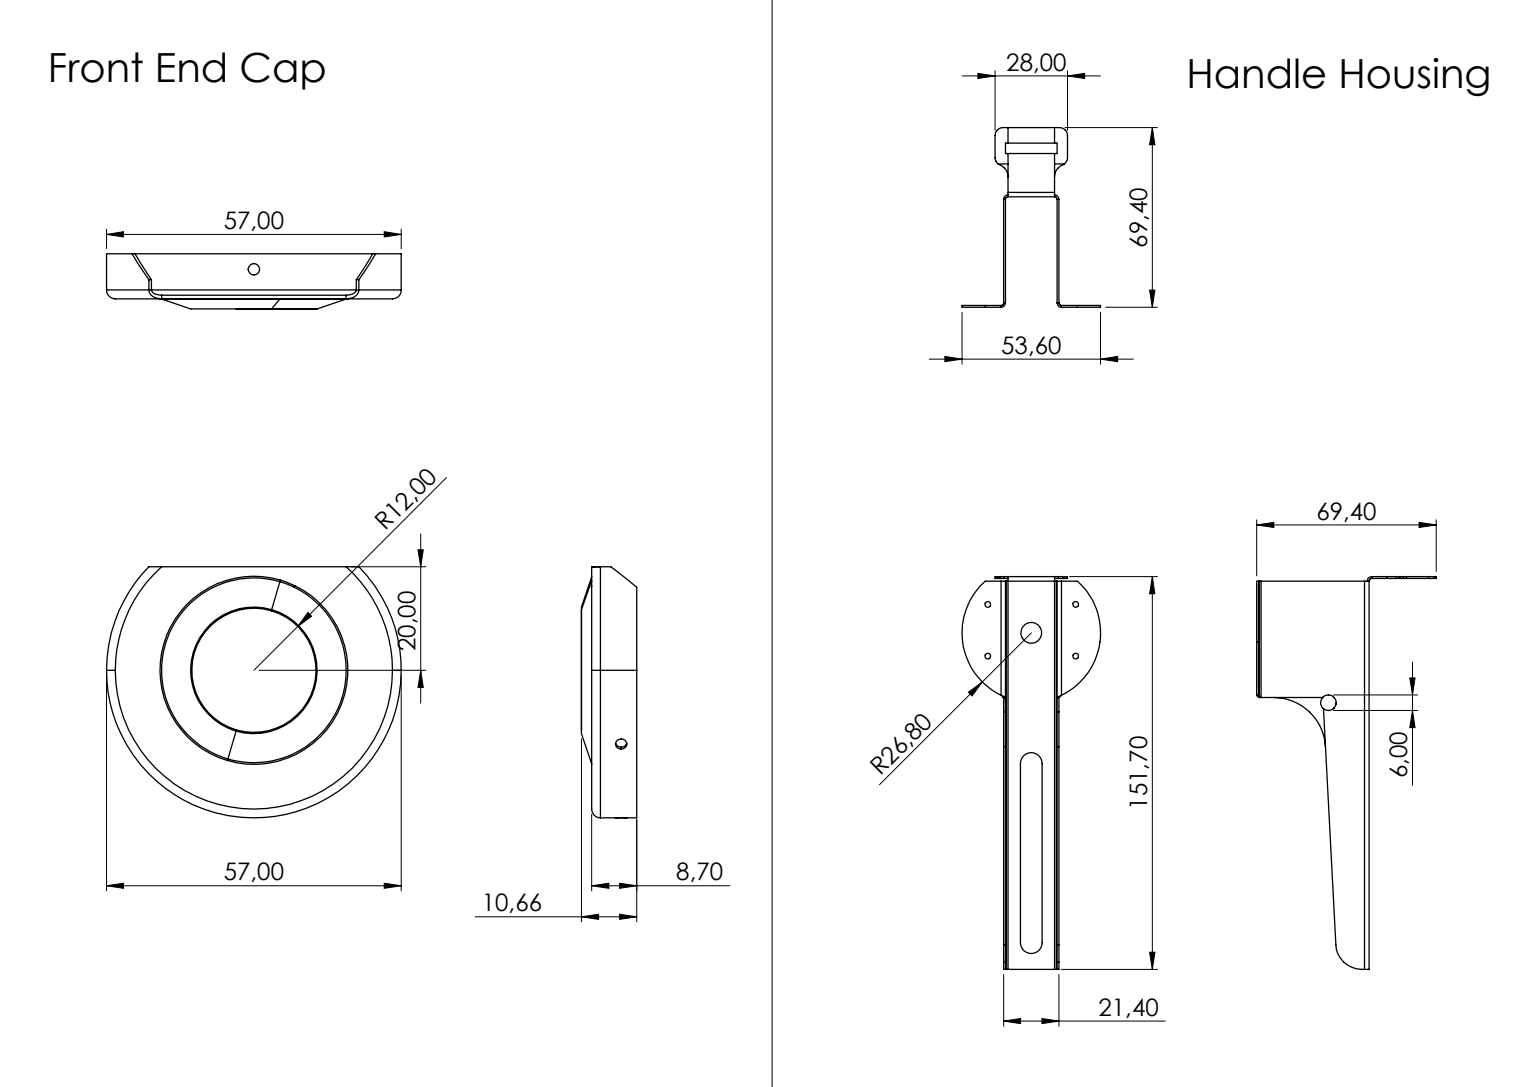
ISO-10303-21;
HEADER;
FILE_DESCRIPTION (('STEP AP214'),
    '1' );
FILE_NAME ('Front End Cap.step',
    '2026-10-06T09:00:30',
    ( '' ),
    ( '' ),
    'SwSTEP 2.0',
    'SolidWorks 2020',
    '' );
FILE_SCHEMA (( 'AUTOMOTIVE_DESIGN' ));
ENDSEC;

DATA;
#20=CARTESIAN_POINT ( 'NONE',  ( -0.8259893079150000261, -28.48844349870000059, 224.2403608809999866 ) ) ;
#22=CARTESIAN_POINT ( 'NONE',  ( 24.25874038310000103, -14.95904359230000047, 225.7601370010000039 ) ) ;
#50=EDGE_CURVE ( 'NONE', #6418, #21281, #18108, .T. ) ;
#55=VERTEX_POINT ( 'NONE', #6316 ) ;
#63=CARTESIAN_POINT ( 'NONE',  ( 24.57933163011563238, -12.98840299560160538, 225.3593307347778136 ) ) ;
#67=CARTESIAN_POINT ( 'NONE',  ( 1.127732790480000080, -28.47784299079999926, 225.0000014190000002 ) ) ;
#70=EDGE_CURVE ( 'NONE', #662, #13739, #1640, .T. ) ;
#83=CARTESIAN_POINT ( 'NONE',  ( 27.71720220739999974, -1.975806291350000238E-11, 229.4485730569999760 ) ) ;
#84=CARTESIAN_POINT ( 'NONE',  ( -11.57541201399999942, -14.20905793120000027, 230.6999999999999886 ) ) ;
#86=CARTESIAN_POINT ( 'NONE',  ( 25.26810488179999936, 12.77004255139999955, 229.0000000000000000 ) ) ;
#91=CARTESIAN_POINT ( 'NONE',  ( 20.67177784749999958, 17.22892977999999786, 230.6999999999999886 ) ) ;
#104=CARTESIAN_POINT ( 'NONE',  ( 24.55806919409999978, -14.46257963250000067, 223.9201486480000085 ) ) ;
#111=CARTESIAN_POINT ( 'NONE',  ( 24.34123158960000310, -14.82477075290000101, 225.9012998019999827 ) ) ;
#112=CARTESIAN_POINT ( 'NONE',  ( -12.01652311039999965, 1.520041121179999788, 231.9999989789999972 ) ) ;
#117=CARTESIAN_POINT ( 'NONE',  ( 24.40260331739102639, -13.31784478726558163, 224.1134674150510477 ) ) ;
#138=CARTESIAN_POINT ( 'NONE',  ( 28.49999999979999998, 4.443028818220000176, 229.0000000000000000 ) ) ;
#140=CARTESIAN_POINT ( 'NONE',  ( 5.010073463369999480, 11.17224087250000153, 232.6627648150000027 ) ) ;
#199=ORIENTED_EDGE ( 'NONE', *, *, #6289, .F. ) ;
#200=CARTESIAN_POINT ( 'NONE',  ( 25.11738521000000190, -13.46751580659999981, 225.6806823370000075 ) ) ;
#209=CARTESIAN_POINT ( 'NONE',  ( -5.361385120510000490, 31.61859227569999931, 222.0000000000000000 ) ) ;
#217=CARTESIAN_POINT ( 'NONE',  ( 24.50095082274352265, -13.13603084652294051, 225.6822660555842219 ) ) ;
#235=CARTESIAN_POINT ( 'NONE',  ( 21.99374050320000151, 17.63454380109999775, 229.1414208810000162 ) ) ;
#239=CARTESIAN_POINT ( 'NONE',  ( 22.83443070970000122, 16.43389729289999934, 229.0000000010000178 ) ) ;
#270=CARTESIAN_POINT ( 'NONE',  ( -26.95773186790000153, 8.656139628340000058, 223.3999999999999773 ) ) ;
#280=CARTESIAN_POINT ( 'NONE',  ( 23.65332633301680687, -14.60697862033088512, 225.7326966119605061 ) ) ;
#285=ORIENTED_EDGE ( 'NONE', *, *, #4802, .T. ) ;
#289=CARTESIAN_POINT ( 'NONE',  ( -24.87138426050000106, -13.91768300640000078, 223.9574921340000060 ) ) ;
#292=CARTESIAN_POINT ( 'NONE',  ( 24.30716200859999887, -13.49132717699999873, 226.0027513979999867 ) ) ;
#302=CARTESIAN_POINT ( 'NONE',  ( 8.575788938069999645, 8.809323376420000073, 232.6627648150000027 ) ) ;
#306=CARTESIAN_POINT ( 'NONE',  ( 28.49999999970000175, -7.466149220240000162, 229.2404163060000144 ) ) ;
#319=CARTESIAN_POINT ( 'NONE',  ( -24.34385441500000269, 13.50419739129999996, 229.9172023120000006 ) ) ;
#333=CARTESIAN_POINT ( 'NONE',  ( -0.07056952541350000607, -28.50017087330000010, 223.9013489249999793 ) ) ;
#354=B_SPLINE_SURFACE_WITH_KNOTS ( 'NONE', 5, 1, ( 
 ( #10886, #5534 ),
 ( #25047, #15138 ),
 ( #29454, #22387 ),
 ( #22540, #832 ),
 ( #10575, #22684 ),
 ( #7887, #24739 ) ),
 .UNSPECIFIED., .F., .F., .F.,
 ( 6, 6 ),
 ( 2, 2 ),
 ( 0.000000000000000000, 2.000000000000000000 ),
 ( 4.440892098500000003E-16, 0.7000000000030000002 ),
 .UNSPECIFIED. ) ;
#379=ORIENTED_EDGE ( 'NONE', *, *, #13979, .T. ) ;
#392=CARTESIAN_POINT ( 'NONE',  ( 25.84472112319999937, 9.051226241580000220, 230.0000000000000000 ) ) ;
#406=ORIENTED_EDGE ( 'NONE', *, *, #23149, .F. ) ;
#426=CARTESIAN_POINT ( 'NONE',  ( -7.523368333400000552, -9.723541495030000092, 232.6627643349999914 ) ) ;
#429=CARTESIAN_POINT ( 'NONE',  ( -6.304462755850305911, -10.33059293845434645, 232.0000000000046043 ) ) ;
#433=B_SPLINE_CURVE_WITH_KNOTS ( 'NONE', 5,
 ( #4051, #25135, #25459, #5930, #17879, #25619 ),
 .UNSPECIFIED., .F., .F.,
 ( 6, 6 ),
 ( -7.000000000120000010, -4.999999893120000038 ),
 .UNSPECIFIED. ) ;
#444=CARTESIAN_POINT ( 'NONE',  ( -24.26052213770000066, -13.57583965319999919, 223.9574921340000060 ) ) ;
#453=VERTEX_POINT ( 'NONE', #9877 ) ;
#456=CARTESIAN_POINT ( 'NONE',  ( -24.82465127917437542, -14.00098045660550916, 223.9261769685532784 ) ) ;
#457=CARTESIAN_POINT ( 'NONE',  ( 10.59650700230000098, -5.774382186429999564, 231.9999991140000191 ) ) ;
#466=ADVANCED_FACE ( 'NONE', ( #21379 ), #11165, .F. ) ;
#477=CARTESIAN_POINT ( 'NONE',  ( -26.13021838950000131, 9.136631768579999147, 229.9751247030000059 ) ) ;
#484=ORIENTED_EDGE ( 'NONE', *, *, #3647, .F. ) ;
#488=CARTESIAN_POINT ( 'NONE',  ( 18.64708650441101767, 19.99999271436163539, 230.6104614892431073 ) ) ;
#495=CARTESIAN_POINT ( 'NONE',  ( -20.30396347049999761, 20.00000000670000233, 227.0000000000000000 ) ) ;
#508=CARTESIAN_POINT ( 'NONE',  ( 1.015231355570000105, -28.48218680760000154, 225.5064715119999903 ) ) ;
#529=FACE_OUTER_BOUND ( 'NONE', #18862, .T. ) ;
#532=EDGE_CURVE ( 'NONE', #10448, #2003, #10192, .T. ) ;
#543=CARTESIAN_POINT ( 'NONE',  ( -0.9721910944845530977, -28.48371442619422567, 224.4394323450521540 ) ) ;
#551=CARTESIAN_POINT ( 'NONE',  ( 26.78508784419999955, 9.380747199480000020, 229.2930777859999978 ) ) ;
#552=CARTESIAN_POINT ( 'NONE',  ( -10.87631678760000042, 14.78838196149999895, 230.6999999999999886 ) ) ;
#560=ADVANCED_FACE ( 'NONE', ( #602, #27628 ), #17709, .F. ) ;
#595=CARTESIAN_POINT ( 'NONE',  ( 24.19477113890000197, -13.69187437440000110, 226.0798554400000171 ) ) ;
#602=FACE_BOUND ( 'NONE', #30223, .T. ) ;
#606=CARTESIAN_POINT ( 'NONE',  ( 11.05434102880000147, 5.380509146490000560, 232.6627648150000027 ) ) ;
#627=CARTESIAN_POINT ( 'NONE',  ( -18.03440174900000059, 20.21871556809999859, 229.9751246760000072 ) ) ;
#630=B_SPLINE_CURVE_WITH_KNOTS ( 'NONE', 1,
 ( #19801, #8283 ),
 .UNSPECIFIED., .F., .F.,
 ( 2, 2 ),
 ( -2.557291473029999731E-06, 0.7000000000009999335 ),
 .UNSPECIFIED. ) ;
#631=B_SPLINE_CURVE_WITH_KNOTS ( 'NONE', 5,
 ( #31112, #6871, #7037, #18836, #26396, #16473, #11758, #23732, #2168 ),
 .UNSPECIFIED., .F., .F.,
 ( 6, 3, 6 ),
 ( 8.011061266649999624, 8.811732102769999742, 9.612402938880000747 ),
 .UNSPECIFIED. ) ;
#662=VERTEX_POINT ( 'NONE', #3400 ) ;
#692=CARTESIAN_POINT ( 'NONE',  ( -0.8418772534729759283, -28.48787735128006560, 224.2649303555695326 ) ) ;
#738=SURFACE_STYLE_USAGE ( .BOTH. , #10017 ) ;
#742=LINE ( 'NONE', #24800, #23892 ) ;
#755=CARTESIAN_POINT ( 'NONE',  ( -23.69119896560000171, -20.94188573509999785, 229.0000000000000000 ) ) ;
#776=CARTESIAN_POINT ( 'NONE',  ( -27.79999999999999716, -2.358414161360000020E-11, 229.1414213560000235 ) ) ;
#780=CIRCLE ( 'NONE', #14848, 17.84349269770000035 ) ;
#803=DIRECTION ( 'NONE',  ( 0.4353787270609792981, 0.9002473904559574747, 0.000000000000000000 ) ) ;
#804=B_SPLINE_CURVE_WITH_KNOTS ( 'NONE', 5,
 ( #6023, #8370, #8687, #25708, #20976, #25393 ),
 .UNSPECIFIED., .F., .F.,
 ( 6, 6 ),
 ( -7.118285296629999870, 0.000000000000000000 ),
 .UNSPECIFIED. ) ;
#809=CARTESIAN_POINT ( 'NONE',  ( -28.50000000000000000, -4.181985830669999980E-14, 229.2404163060000144 ) ) ;
#823=ORIENTED_EDGE ( 'NONE', *, *, #1132, .F. ) ;
#827=CARTESIAN_POINT ( 'NONE',  ( 133283.2432719999924, 454259.0741890000063, -160669.1380380000046 ) ) ;
#832=CARTESIAN_POINT ( 'NONE',  ( -19.80526803560000104, 19.50877411510000314, 227.8000000000000114 ) ) ;
#843=CARTESIAN_POINT ( 'NONE',  ( -28.49999999979999998, 4.805538726630000923, 229.2404163060000144 ) ) ;
#880=CARTESIAN_POINT ( 'NONE',  ( -7.131609927916050751, 9.777910867662733096, 232.0000000000051159 ) ) ;
#889=CARTESIAN_POINT ( 'NONE',  ( 23.69119887989999995, 20.94188554249999967, 222.0000000000000000 ) ) ;
#910=CARTESIAN_POINT ( 'NONE',  ( -24.75565187725877081, -14.12271910255536689, 223.9000014190000059 ) ) ;
#951=CARTESIAN_POINT ( 'NONE',  ( -22.97554861169999896, 15.65134970780000145, 222.0000000000000000 ) ) ;
#964=CARTESIAN_POINT ( 'NONE',  ( 19.80538173989999962, 19.50875420239999869, 229.0000000000000000 ) ) ;
#979=VERTEX_POINT ( 'NONE', #23204 ) ;
#982=DIRECTION ( 'NONE',  ( 1.000000000000000000, 0.000000000000000000, 0.000000000000000000 ) ) ;
#994=CARTESIAN_POINT ( 'NONE',  ( 25.22036945370000183, -13.27344566769999901, 224.7916409239999780 ) ) ;
#996=CARTESIAN_POINT ( 'NONE',  ( -18.97091445539999910, 21.26865671750000075, 229.0000000000000000 ) ) ;
#1002=CARTESIAN_POINT ( 'NONE',  ( 3.184793790070000075, -18.07879718899999943, 230.6999999999999886 ) ) ;
#1022=CARTESIAN_POINT ( 'NONE',  ( -28.23997156040000078, -4.869988983339999855, 222.0000000000000000 ) ) ;
#1024=EDGE_CURVE ( 'NONE', #18614, #4760, #2033, .T. ) ;
#1030=CARTESIAN_POINT ( 'NONE',  ( 25.20859211119999799, -13.29584934979999922, 224.6894611300000122 ) ) ;
#1032=CARTESIAN_POINT ( 'NONE',  ( -28.50000000000000000, 4.194175870809999815E-15, 222.0000000000000000 ) ) ;
#1041=CARTESIAN_POINT ( 'NONE',  ( 27.98881761119999823, 6.827871301039999175, 222.0000000000000000 ) ) ;
#1049=CARTESIAN_POINT ( 'NONE',  ( 18.65395304217032901, 19.99999294228678792, 230.6088730870111476 ) ) ;
#1052=EDGE_CURVE ( 'NONE', #12887, #10989, #2292, .T. ) ;
#1058=CARTESIAN_POINT ( 'NONE',  ( -24.68204616399999907, -14.25020164319999871, 223.9000014189999774 ) ) ;
#1061=CARTESIAN_POINT ( 'NONE',  ( -0.1033151399490000039, -27.80006701330000141, 223.9040511909999793 ) ) ;
#1075=CARTESIAN_POINT ( 'NONE',  ( -17.83931601680000156, 20.00000000000000000, 230.7000111870000012 ) ) ;
#1078=ORIENTED_EDGE ( 'NONE', *, *, #22876, .T. ) ;
#1102=CARTESIAN_POINT ( 'NONE',  ( -24.40276494859777046, -13.31831424753606008, 225.8868154035638156 ) ) ;
#1118=CARTESIAN_POINT ( 'NONE',  ( -24.46845037339999962, -13.19716075180000026, 224.2397332909999932 ) ) ;
#1125=CARTESIAN_POINT ( 'NONE',  ( 26.32519403849999762, 9.219495376610002069, 230.6577119970000069 ) ) ;
#1132=EDGE_CURVE ( 'NONE', #6418, #6498, #7888, .T. ) ;
#1134=ORIENTED_EDGE ( 'NONE', *, *, #23818, .T. ) ;
#1140=CARTESIAN_POINT ( 'NONE',  ( -28.35924375250000296, -1.021553995729999846E-14, 229.7625741969999922 ) ) ;
#1143=CARTESIAN_POINT ( 'NONE',  ( -1.854631282479999976, -18.18682133599999773, 230.6999999999999886 ) ) ;
#1145=ORIENTED_EDGE ( 'NONE', *, *, #22578, .F. ) ;
#1157=ORIENTED_EDGE ( 'NONE', *, *, #15638, .T. ) ;
#1204=VERTEX_POINT ( 'NONE', #12261 ) ;
#1205=CARTESIAN_POINT ( 'NONE',  ( 19.01242865374335267, 20.00033489853029778, 230.5035276049833044 ) ) ;
#1228=ADVANCED_FACE ( 'NONE', ( #4721 ), #23930, .F. ) ;
#1232=CARTESIAN_POINT ( 'NONE',  ( -20.01708959866950366, 19.99999743978112932, 229.8069797309569822 ) ) ;
#1241=EDGE_LOOP ( 'NONE', ( #8778, #2335, #4602, #30893 ) ) ;
#1266=CARTESIAN_POINT ( 'NONE',  ( 0.4821455018050000429, -28.49635764770000179, 226.0025203910000187 ) ) ;
#1270=CARTESIAN_POINT ( 'NONE',  ( 0.2462945485190000117, -28.49939181899999951, 223.9202078600000050 ) ) ;
#1273=VERTEX_POINT ( 'NONE', #28778 ) ;
#1277=ORIENTED_EDGE ( 'NONE', *, *, #11164, .F. ) ;
#1287=CARTESIAN_POINT ( 'NONE',  ( -1.087696845100000198, -27.77899371300000197, 224.7918862260000026 ) ) ;
#1288=PRODUCT ( 'Front End Cap', 'Front End Cap', '', ( #16022 ) ) ;
#1303=CARTESIAN_POINT ( 'NONE',  ( -24.15788560609999891, 13.40103774969999861, 230.6999999999999886 ) ) ;
#1304=DIRECTION ( 'NONE',  ( 0.000000000000000000, 0.000000000000000000, -1.000000000000000000 ) ) ;
#1307=CARTESIAN_POINT ( 'NONE',  ( 18.42247763970000207, -19.87503982779999845, 230.6999999999999886 ) ) ;
#1327=CARTESIAN_POINT ( 'NONE',  ( -23.10935684520000066, -20.42749692159999952, 229.1414198580000061 ) ) ;
#1337=CARTESIAN_POINT ( 'NONE',  ( 19.80537707610000098, 19.50874960790000046, 229.0739602739999725 ) ) ;
#1339=CARTESIAN_POINT ( 'NONE',  ( 24.71695093370000151, -14.18891100779999981, 223.9013457789999961 ) ) ;
#1350=CARTESIAN_POINT ( 'NONE',  ( 26.95545381250000361, 8.667969360499998999, 227.5999999999999943 ) ) ;
#1357=( NAMED_UNIT ( * ) PLANE_ANGLE_UNIT ( ) SI_UNIT ( $, .RADIAN. ) );
#1362=CARTESIAN_POINT ( 'NONE',  ( 18.77987097257140903, 20.00007305761831589, 230.5773074074296005 ) ) ;
#1381=CARTESIAN_POINT ( 'NONE',  ( -24.10559463919999956, -15.20494734660000091, 225.2084356629999888 ) ) ;
#1390=CARTESIAN_POINT ( 'NONE',  ( -20.12793915297035952, 19.99999059665350387, 229.6434139119940312 ) ) ;
#1424=CARTESIAN_POINT ( 'NONE',  ( 20.30405755279999980, 20.00000000000000000, 227.3999999149999951 ) ) ;
#1429=EDGE_LOOP ( 'NONE', ( #7369, #15757, #8978, #15625 ) ) ;
#1434=CARTESIAN_POINT ( 'NONE',  ( -24.55564696219999732, -13.03410599059999875, 224.4928762930000232 ) ) ;
#1455=CARTESIAN_POINT ( 'NONE',  ( -0.2462327729630000017, -28.49941772390000239, 226.0797932899999978 ) ) ;
#1461=CARTESIAN_POINT ( 'NONE',  ( -26.80000000000000071, -8.704148513059999178E-14, 230.6999999999999886 ) ) ;
#1463=CARTESIAN_POINT ( 'NONE',  ( -27.56257419730000180, -2.228452907019999617E-14, 230.5592437530000041 ) ) ;
#1466=CIRCLE ( 'NONE', #5956, 0.9999999999999981126 ) ;
#1467=CARTESIAN_POINT ( 'NONE',  ( -23.10935684540000068, -20.42749692129999772, 222.0000000000000000 ) ) ;
#1468=CARTESIAN_POINT ( 'NONE',  ( 26.80000000069999899, -1.877389046380000037, 230.6999999999999886 ) ) ;
#1490=CARTESIAN_POINT ( 'NONE',  ( 5.229687933750000184, -30.84198039029999805, 229.1414219810000077 ) ) ;
#1513=CARTESIAN_POINT ( 'NONE',  ( -26.05511412830000140, 14.93229958979999950, 222.0000000000000000 ) ) ;
#1523=CARTESIAN_POINT ( 'NONE',  ( 19.58403526555239793, 20.00013581975909815, 230.2127468032437889 ) ) ;
#1601=CARTESIAN_POINT ( 'NONE',  ( -25.17394274020000111, -13.36230406159999973, 225.5071265450000055 ) ) ;
#1606=CARTESIAN_POINT ( 'NONE',  ( -1.127665019380000189, -28.47796022459999676, 225.0000014190000002 ) ) ;
#1612=CARTESIAN_POINT ( 'NONE',  ( 24.71695093370000151, -14.18891100779999981, 223.9013457789999961 ) ) ;
#1615=CARTESIAN_POINT ( 'NONE',  ( -24.62906106470000012, -14.34164290000000008, 226.0959707279999975 ) ) ;
#1616=B_SPLINE_CURVE_WITH_KNOTS ( 'NONE', 1,
 ( #9249, #23599 ),
 .UNSPECIFIED., .F., .F.,
 ( 2, 2 ),
 ( -2.557302930970000000E-06, 0.7000000000009999335 ),
 .UNSPECIFIED. ) ;
#1618=CARTESIAN_POINT ( 'NONE',  ( 9.315522638039999137, 15.62494945029999904, 230.6999999999999886 ) ) ;
#1626=CARTESIAN_POINT ( 'NONE',  ( 28.49999999990000177, 3.413935693800000060, 222.0000000000000000 ) ) ;
#1630=CARTESIAN_POINT ( 'NONE',  ( -24.87138426050000106, -13.91768300640000078, 226.0425107039999943 ) ) ;
#1640=B_SPLINE_CURVE_WITH_KNOTS ( 'NONE', 1,
 ( #22386, #24898 ),
 .UNSPECIFIED., .F., .F.,
 ( 2, 2 ),
 ( -9.355471259890000464E-07, 0.7003637394550000783 ),
 .UNSPECIFIED. ) ;
#1642=CARTESIAN_POINT ( 'NONE',  ( 5.068184391690000012, -29.88946390619999960, 230.0000000000000000 ) ) ;
#1644=CARTESIAN_POINT ( 'NONE',  ( -18.43841600009999837, -21.14227905559999954, 222.0000000000000000 ) ) ;
#1676=CARTESIAN_POINT ( 'NONE',  ( -18.31101975560000028, 19.88193351600000014, 229.9783743860000129 ) ) ;
#1691=CARTESIAN_POINT ( 'NONE',  ( 1.379841223609999723, 12.21656123380000025, 232.6627643349999914 ) ) ;
#1692=CARTESIAN_POINT ( 'NONE',  ( -1.776356839399999804E-15, -1.776356839399999804E-15, 230.0000000000000000 ) ) ;
#1703=CARTESIAN_POINT ( 'NONE',  ( -23.62732472759999780, -14.64974168890000072, 224.3191706570000292 ) ) ;
#1720=CARTESIAN_POINT ( 'NONE',  ( -20.30396346370000060, 20.00000000000000000, 227.0000000000000000 ) ) ;
#1723=CARTESIAN_POINT ( 'NONE',  ( 20.08301454169999900, -20.21156784769999959, 230.6999999999999886 ) ) ;
#1732=CARTESIAN_POINT ( 'NONE',  ( 0.3737937747629999641, -27.79795631750000240, 223.9576737099999946 ) ) ;
#1733=( GEOMETRIC_REPRESENTATION_CONTEXT ( 3 ) GLOBAL_UNCERTAINTY_ASSIGNED_CONTEXT ( ( #11892 ) ) GLOBAL_UNIT_ASSIGNED_CONTEXT ( ( #10483, #15192, #15352 ) ) REPRESENTATION_CONTEXT ( 'NONE', 'WORKASPACE' ) );
#1744=ORIENTED_EDGE ( 'NONE', *, *, #15831, .F. ) ;
#1759=CARTESIAN_POINT ( 'NONE',  ( -25.08454981450000076, -13.52946590100000179, 225.7602695480000250 ) ) ;
#1775=CARTESIAN_POINT ( 'NONE',  ( -24.84642331740000287, 12.90500083959999955, 222.0000000000000000 ) ) ;
#1790=CARTESIAN_POINT ( 'NONE',  ( -25.22658730140000216, -13.26242337740000110, 225.0000014190000002 ) ) ;
#1795=DIRECTION ( 'NONE',  ( 0.2815395311429191860, 0.9595496299847263710, 0.000000000000000000 ) ) ;
#1801=CARTESIAN_POINT ( 'NONE',  ( 27.71720220710000149, -7.261079543219999266, 229.4485730569999760 ) ) ;
#1803=CARTESIAN_POINT ( 'NONE',  ( 1.127732790480000080, -28.47784299079999926, 225.0000014190000002 ) ) ;
#1807=ORIENTED_EDGE ( 'NONE', *, *, #18680, .F. ) ;
#1812=CARTESIAN_POINT ( 'NONE',  ( 9.961462855526637128, 7.265485266898056516, 232.6627635728646908 ) ) ;
#1817=CARTESIAN_POINT ( 'NONE',  ( 1.115119965759999943, -28.47834310740000063, 225.2081038119999903 ) ) ;
#1820=CARTESIAN_POINT ( 'NONE',  ( 27.79999999999999716, -2.352606998100000196E-11, 229.0000000000000000 ) ) ;
#1846=CARTESIAN_POINT ( 'NONE',  ( 20.30406631279999985, 20.00000862929999812, 229.1257344590000002 ) ) ;
#1849=CARTESIAN_POINT ( 'NONE',  ( -1.089818731930000117, -28.47945802909999813, 225.3102023309999993 ) ) ;
#1860=B_SPLINE_CURVE_WITH_KNOTS ( 'NONE', 1,
 ( #6195, #25409 ),
 .UNSPECIFIED., .F., .F.,
 ( 2, 2 ),
 ( -0.7000000000030000002, -4.440892098500626162E-16 ),
 .UNSPECIFIED. ) ;
#1872=CIRCLE ( 'NONE', #11449, 17.84349269770000035 ) ;
#1873=FACE_OUTER_BOUND ( 'NONE', #20051, .T. ) ;
#1878=CARTESIAN_POINT ( 'NONE',  ( -22.47789033090000288, -19.86937924559999757, 230.6999999999999886 ) ) ;
#1884=CARTESIAN_POINT ( 'NONE',  ( 0.03533597110129999691, -28.50021994999999819, 223.9000014189999774 ) ) ;
#1888=B_SPLINE_SURFACE_WITH_KNOTS ( 'NONE', 5, 1, ( 
 ( #25832, #30398 ),
 ( #13549, #23631 ),
 ( #20632, #9290 ),
 ( #4270, #11190 ),
 ( #1601, #11042 ),
 ( #28331, #20789 ),
 ( #1759, #8979 ),
 ( #6780, #27702 ),
 ( #21106, #6149 ),
 ( #8820, #2066 ),
 ( #25984, #16068 ),
 ( #15748, #4421 ),
 ( #25677, #23311 ),
 ( #11657, #25361 ),
 ( #11349, #22998 ) ),
 .UNSPECIFIED., .F., .F., .F.,
 ( 6, 3, 3, 3, 6 ),
 ( 2, 2 ),
 ( 0.000000000000000000, 0.5239049114870000246, 1.047809822970000138, 1.571714734459999985, 1.746349704960000082 ),
 ( -0.7000000000009999335, 2.557517344899999924E-06 ),
 .UNSPECIFIED. ) ;
#1898=CARTESIAN_POINT ( 'NONE',  ( -24.19505510210000310, -13.69211658319999891, 223.9201349309999785 ) ) ;
#1906=CARTESIAN_POINT ( 'NONE',  ( 21.20256267760000313, 17.00023892710000339, 230.6999999999999886 ) ) ;
#1920=ORIENTED_EDGE ( 'NONE', *, *, #20595, .F. ) ;
#1952=CARTESIAN_POINT ( 'NONE',  ( 25.39242439670000095, -14.55250846959999933, 229.2930774670000176 ) ) ;
#1966=CARTESIAN_POINT ( 'NONE',  ( 3.441895497200000431, 11.73074891959999988, 232.6627635220000059 ) ) ;
#1970=CARTESIAN_POINT ( 'NONE',  ( -23.08673860280000056, 15.48734418929999990, 222.0000000000000000 ) ) ;
#1993=CARTESIAN_POINT ( 'NONE',  ( -17.83931601680000156, 20.00000000000000000, 230.7000111870000012 ) ) ;
#2003=VERTEX_POINT ( 'NONE', #13269 ) ;
#2006=CARTESIAN_POINT ( 'NONE',  ( 19.65673127730000402, 20.00000654480000151, 230.1824637990000042 ) ) ;
#2007=CARTESIAN_POINT ( 'NONE',  ( -25.27355175290000133, 12.75978488059999805, 227.5999999999999943 ) ) ;
#2033=CIRCLE ( 'NONE', #14094, 18.16530045500000057 ) ;
#2034=CARTESIAN_POINT ( 'NONE',  ( -5.056117937459999823, -11.13261400500000065, 232.6627648150000027 ) ) ;
#2038=CARTESIAN_POINT ( 'NONE',  ( 5.041582825300000792, -29.73257086209999756, 230.6999999999999886 ) ) ;
#2045=CARTESIAN_POINT ( 'NONE',  ( -24.30742244220000003, -13.49161940279999961, 223.9971936000000028 ) ) ;
#2063=CARTESIAN_POINT ( 'NONE',  ( -0.2402207101440000103, -27.79943747540000132, 223.9202095490000204 ) ) ;
#2064=ADVANCED_BREP_SHAPE_REPRESENTATION ( '', ( #21535, #17722 ), #25295 ) ;
#2066=CARTESIAN_POINT ( 'NONE',  ( -24.26052213759999887, -13.57583965329999920, 226.0425107039999943 ) ) ;
#2073=CARTESIAN_POINT ( 'NONE',  ( -18.92356980859999993, 19.72862807099999927, 229.8505673220000176 ) ) ;
#2090=CARTESIAN_POINT ( 'NONE',  ( -21.56316276399999765, 17.27952114640000048, 229.9172021830000006 ) ) ;
#2094=CARTESIAN_POINT ( 'NONE',  ( -20.97486481260628821, 18.32139253905734932, 225.3333333333333712 ) ) ;
#2104=CARTESIAN_POINT ( 'NONE',  ( 25.16954019099999940, -14.42477239210000128, 229.7313254700000016 ) ) ;
#2107=CARTESIAN_POINT ( 'NONE',  ( 20.43731315469999998, -19.07003687599999964, 222.0000000000000000 ) ) ;
#2119=FACE_OUTER_BOUND ( 'NONE', #20985, .T. ) ;
#2158=CARTESIAN_POINT ( 'NONE',  ( 1.354415895940000114, 11.99145557159999953, 231.9999989789999972 ) ) ;
#2161=CARTESIAN_POINT ( 'NONE',  ( -0.03526712872429999673, -28.50022367440000082, 226.1000014189999945 ) ) ;
#2168=CARTESIAN_POINT ( 'NONE',  ( -27.79999999999999716, -2.360778239559999931E-11, 229.0000000000000000 ) ) ;
#2173=CARTESIAN_POINT ( 'NONE',  ( -23.50695179570000093, -14.84192241259999889, 224.8957841300000098 ) ) ;
#2175=ORIENTED_EDGE ( 'NONE', *, *, #26586, .T. ) ;
#2187=CARTESIAN_POINT ( 'NONE',  ( -1.674213827660000042, -11.95100239910000006, 231.9999991140000191 ) ) ;
#2193=CARTESIAN_POINT ( 'NONE',  ( 5.361384718760000112, -31.61859215249999977, 229.0000000000000000 ) ) ;
#2195=CARTESIAN_POINT ( 'NONE',  ( -24.09883371379999772, -15.21565466309999870, 225.0000014190000002 ) ) ;
#2205=CARTESIAN_POINT ( 'NONE',  ( -1.419173372180000084E-06, -27.80022181310000207, 223.9000014189999774 ) ) ;
#2222=ORIENTED_EDGE ( 'NONE', *, *, #25739, .F. ) ;
#2223=CARTESIAN_POINT ( 'NONE',  ( 24.10531740749999940, -15.20475527630000023, 225.2083717279999746 ) ) ;
#2252=ORIENTED_EDGE ( 'NONE', *, *, #4611, .T. ) ;
#2265=CARTESIAN_POINT ( 'NONE',  ( 14.09657531829999932, 28.30410039250000054, 222.0000000000000000 ) ) ;
#2266=CARTESIAN_POINT ( 'NONE',  ( -28.50000000000000000, 1.776356839399999922E-14, 222.0000000000000000 ) ) ;
#2271=CARTESIAN_POINT ( 'NONE',  ( 27.79999999999999716, -0.8519342421209999960, 222.0000000000000000 ) ) ;
#2283=AXIS2_PLACEMENT_3D ( 'NONE', #10910, #25547, #27579 ) ;
#2292=B_SPLINE_CURVE_WITH_KNOTS ( 'NONE', 5,
 ( #67, #9334, #4615, #9493, #11858, #19095, #14222, #23828, #28385, #28536, #16718, #28689, #2570, #21304, #7135 ),
 .UNSPECIFIED., .F., .F.,
 ( 6, 3, 3, 3, 6 ),
 ( 0.000000000000000000, 0.2999999999999999889, 0.5999999999977094767, 0.8999999999994273692, 1.000000000000000000 ),
 .UNSPECIFIED. ) ;
#2297=ADVANCED_FACE ( 'NONE', ( #16566 ), #31110, .F. ) ;
#2316=CARTESIAN_POINT ( 'NONE',  ( 24.10531740749999940, -15.20475527630000023, 225.2083717279999746 ) ) ;
#2317=CARTESIAN_POINT ( 'NONE',  ( 0.3163327506049999904, 12.29016939549999954, 232.6627643349999914 ) ) ;
#2319=CARTESIAN_POINT ( 'NONE',  ( -25.27355175290000133, 12.75978488059999805, 223.3999999999999773 ) ) ;
#2321=CARTESIAN_POINT ( 'NONE',  ( -1.087696845100000198, -27.77899371300000197, 225.2081166120000262 ) ) ;
#2335=ORIENTED_EDGE ( 'NONE', *, *, #28038, .F. ) ;
#2342=B_SPLINE_CURVE_WITH_KNOTS ( 'NONE', 1,
 ( #29544, #3262 ),
 .UNSPECIFIED., .F., .F.,
 ( 2, 2 ),
 ( -2.556026448610000073E-06, 0.7000000000009999335 ),
 .UNSPECIFIED. ) ;
#2348=CARTESIAN_POINT ( 'NONE',  ( 24.72074161949999649, -14.16756531389999907, 230.6999999999999886 ) ) ;
#2350=CARTESIAN_POINT ( 'NONE',  ( -24.10559463919999956, -15.20494734660000091, 224.7915671760000009 ) ) ;
#2378=CARTESIAN_POINT ( 'NONE',  ( 24.22190007760000086, -15.01852807150000046, 225.6806946080000102 ) ) ;
#2380=EDGE_CURVE ( 'NONE', #15181, #14446, #21198, .T. ) ;
#2410=ORIENTED_EDGE ( 'NONE', *, *, #6772, .T. ) ;
#2414=CARTESIAN_POINT ( 'NONE',  ( 28.49999999970000175, 10.47094317839999889, 222.0000000000000000 ) ) ;
#2436=CARTESIAN_POINT ( 'NONE',  ( -8.990816569130000602, -15.87649056320000085, 230.6999999999999886 ) ) ;
#2458=CARTESIAN_POINT ( 'NONE',  ( 24.09856112909999837, -15.21545593799999985, 224.8958160969999938 ) ) ;
#2466=CARTESIAN_POINT ( 'NONE',  ( -11.54682818539999900, -3.657609505980000009, 231.9999989789999972 ) ) ;
#2467=CARTESIAN_POINT ( 'NONE',  ( -27.79999999990000248, 4.328052761039999474, 222.0000000000000000 ) ) ;
#2470=CARTESIAN_POINT ( 'NONE',  ( 24.34609883811560849, -13.42112775176797612, 224.0360482199137380 ) ) ;
#2476=CARTESIAN_POINT ( 'NONE',  ( 2.846903786944921855, -11.76275999642770742, 232.0000002394077399 ) ) ;
#2482=ORIENTED_EDGE ( 'NONE', *, *, #14035, .F. ) ;
#2489=CARTESIAN_POINT ( 'NONE',  ( -20.30396346370000060, 20.00000000000000000, 229.0000000000000000 ) ) ;
#2492=CARTESIAN_POINT ( 'NONE',  ( 27.63418825910000010, 8.886057489849999769, 229.0000000000000000 ) ) ;
#2495=CARTESIAN_POINT ( 'NONE',  ( 10.79542655330000045, -5.882779935969999485, 232.6627648150000027 ) ) ;
#2510=CARTESIAN_POINT ( 'NONE',  ( 3.378474373710000034, 11.51459555979999827, 232.0000000000000000 ) ) ;
#2511=CARTESIAN_POINT ( 'NONE',  ( 24.07552309629999954, -13.90001137829999855, 226.1000014189999945 ) ) ;
#2558=ORIENTED_EDGE ( 'NONE', *, *, #18694, .F. ) ;
#2563=CARTESIAN_POINT ( 'NONE',  ( 14.09657531829999932, 28.30410039250000054, 229.0000000000000000 ) ) ;
#2570=CARTESIAN_POINT ( 'NONE',  ( 0.07063658732340000190, -28.50016343120000073, 226.0986540789999992 ) ) ;
#2610=CARTESIAN_POINT ( 'NONE',  ( -10.90668548210000210, -5.673847184790000497, 232.6627643349999914 ) ) ;
#2611=CARTESIAN_POINT ( 'NONE',  ( -22.83911268609999823, 16.42879705509999866, 229.0000000000000000 ) ) ;
#2627=CARTESIAN_POINT ( 'NONE',  ( 0.000000000000000000, 0.000000000000000000, 0.000000000000000000 ) ) ;
#2630=CARTESIAN_POINT ( 'NONE',  ( 25.22625794089999829, -13.26224522399999906, 225.1041818340000020 ) ) ;
#2635=ORIENTED_EDGE ( 'NONE', *, *, #30861, .T. ) ;
#2642=CARTESIAN_POINT ( 'NONE',  ( 3.901012673769999939, 11.36127833220000127, 231.9999991140000191 ) ) ;
#2674=ORIENTED_EDGE ( 'NONE', *, *, #14214, .T. ) ;
#2700=ORIENTED_EDGE ( 'NONE', *, *, #8988, .T. ) ;
#2701=EDGE_CURVE ( 'NONE', #29716, #25525, #15718, .T. ) ;
#2723=CARTESIAN_POINT ( 'NONE',  ( 24.34567703855588761, -13.42188430278006273, 225.9642891784011454 ) ) ;
#2739=CARTESIAN_POINT ( 'NONE',  ( 18.03440925470000167, 20.21871195210000138, 229.9751246720000211 ) ) ;
#2740=CARTESIAN_POINT ( 'NONE',  ( -13.33996868140000025, 12.49968273260000018, 230.6999999999999886 ) ) ;
#2767=CARTESIAN_POINT ( 'NONE',  ( -26.80000000000000071, -7.283063041539999493E-14, 230.0000000000000000 ) ) ;
#2771=CARTESIAN_POINT ( 'NONE',  ( -7.384740713219999364, -9.544372888970000801, 231.9999989789999972 ) ) ;
#2782=CARTESIAN_POINT ( 'NONE',  ( 6.304462385800995605, 10.33059233208346406, 232.0000002394077114 ) ) ;
#2787=CARTESIAN_POINT ( 'NONE',  ( 24.09856112909268688, -15.21545593799569751, 224.8524796740992144 ) ) ;
#2788=EDGE_CURVE ( 'NONE', #16560, #17135, #2973, .T. ) ;
#2816=CARTESIAN_POINT ( 'NONE',  ( -24.59646680460000212, 13.64432696080000085, 229.7313261780000175 ) ) ;
#2828=CARTESIAN_POINT ( 'NONE',  ( 20.05330963473244310, 19.99997410271232923, 229.7574610911009643 ) ) ;
#2836=CARTESIAN_POINT ( 'NONE',  ( -23.65375779729673056, -14.60692596462244985, 224.2670087215145998 ) ) ;
#2839=CARTESIAN_POINT ( 'NONE',  ( 0.2829221443748314302, -27.79908343203750576, 226.0728295493879614 ) ) ;
#2849=B_SPLINE_SURFACE_WITH_KNOTS ( 'NONE', 5, 1, ( 
 ( #3454, #15271 ),
 ( #1424, #25339 ),
 ( #8481, #20767 ),
 ( #15567, #20296 ),
 ( #20452, #30049 ),
 ( #13056, #964 ) ),
 .UNSPECIFIED., .F., .F., .F.,
 ( 6, 6 ),
 ( 2, 2 ),
 ( 4.999999893120000038, 7.000000000120000010 ),
 ( -5.329070518200000398E-15, 0.7000000000219999130 ),
 .UNSPECIFIED. ) ;
#2883=CARTESIAN_POINT ( 'NONE',  ( 27.79999999470000205, -2.355808389319999976E-11, 222.0000000000000000 ) ) ;
#2887=CARTESIAN_POINT ( 'NONE',  ( 21.97405983070000346, 17.61876539540000053, 229.2930768050000268 ) ) ;
#2892=EDGE_CURVE ( 'NONE', #29947, #18419, #1860, .T. ) ;
#2903=EDGE_CURVE ( 'NONE', #27611, #12887, #8583, .T. ) ;
#2912=AXIS2_PLACEMENT_3D ( 'NONE', #8307, #25003, #27364 ) ;
#2918=CARTESIAN_POINT ( 'NONE',  ( -1.836086644060000106, -11.92016782080000148, 231.9999989789999972 ) ) ;
#2927=CARTESIAN_POINT ( 'NONE',  ( -17.83931601609999973, 20.00000000000000000, 230.0000000010000178 ) ) ;
#2931=CARTESIAN_POINT ( 'NONE',  ( -3.378474373710000034, -11.51459555979999827, 232.0000000000000000 ) ) ;
#2936=CARTESIAN_POINT ( 'NONE',  ( -24.91946588839999777, -13.83134141909999926, 223.9971936000000028 ) ) ;
#2937=CARTESIAN_POINT ( 'NONE',  ( 25.00924755590000004, -13.66774365989999929, 225.9012973829999851 ) ) ;
#2946=DIRECTION ( 'NONE',  ( 1.000000000000000000, 0.000000000000000000, 0.000000000000000000 ) ) ;
#2949=CARTESIAN_POINT ( 'NONE',  ( 4.497730495419999919, 11.38816151149999989, 232.6627648150000027 ) ) ;
#2953=CARTESIAN_POINT ( 'NONE',  ( 27.56257419720000357, -7.220571643900000502, 230.5592437530000041 ) ) ;
#2971=CARTESIAN_POINT ( 'NONE',  ( -24.20493445730000204, 13.42713550600000083, 229.9751247330000012 ) ) ;
#2973=B_SPLINE_CURVE_WITH_KNOTS ( 'NONE', 5,
 ( #11116, #27950, #13630, #1676, #27784, #16452, #13783, #6231, #11583, #15840, #20879, #18653, #18504, #28416, #30311 ),
 .UNSPECIFIED., .F., .F.,
 ( 6, 3, 3, 3, 6 ),
 ( 0.000000000000000000, 0.2999999999986154298, 0.6000000000006923129, 0.7999999999996538769, 1.000000000000000000 ),
 .UNSPECIFIED. ) ;
#2986=CARTESIAN_POINT ( 'NONE',  ( 24.34123158960000310, -14.82477075290000101, 225.9012998019999827 ) ) ;
#3002=CARTESIAN_POINT ( 'NONE',  ( 0.3832430167449999980, -28.49789927060000139, 226.0423291289999952 ) ) ;
#3018=CARTESIAN_POINT ( 'NONE',  ( 25.41683733030000170, 14.11523383709999990, 229.4982322489999831 ) ) ;
#3039=CARTESIAN_POINT ( 'NONE',  ( -17.91346663230000047, 3.647998880369999863, 230.6999999999999886 ) ) ;
#3065=ORIENTED_EDGE ( 'NONE', *, *, #7121, .T. ) ;
#3068=CARTESIAN_POINT ( 'NONE',  ( -11.53315104089999998, 3.551884179650000029, 231.9999989789999972 ) ) ;
#3098=CARTESIAN_POINT ( 'NONE',  ( 8.011542175009999767, -9.024668540559998675, 231.9999991140000191 ) ) ;
#3105=EDGE_CURVE ( 'NONE', #8755, #29481, #4231, .T. ) ;
#3147=CARTESIAN_POINT ( 'NONE',  ( -24.49868928475705943, -13.14068576356688922, 225.6775953917510265 ) ) ;
#3187=CARTESIAN_POINT ( 'NONE',  ( -25.46187654339999895, 14.12439703469999941, 229.2404163060000144 ) ) ;
#3190=CARTESIAN_POINT ( 'NONE',  ( 21.99374050320000151, 17.63454380079999950, 229.0000000010000178 ) ) ;
#3205=ORIENTED_EDGE ( 'NONE', *, *, #22083, .F. ) ;
#3210=FACE_OUTER_BOUND ( 'NONE', #21529, .T. ) ;
#3217=CARTESIAN_POINT ( 'NONE',  ( 19.29843289230000281, 19.63498672150000246, 229.6955567279999855 ) ) ;
#3224=AXIS2_PLACEMENT_3D ( 'NONE', #12743, #22356, #803 ) ;
#3230=CARTESIAN_POINT ( 'NONE',  ( -23.94309786560000219, 13.28188914049999880, 230.0000000000000000 ) ) ;
#3250=DIRECTION ( 'NONE',  ( 0.000000000000000000, 0.000000000000000000, 1.000000000000000000 ) ) ;
#3262=CARTESIAN_POINT ( 'NONE',  ( 24.68173674080000168, -14.25001227039999918, 226.1000014189999945 ) ) ;
#3268=CARTESIAN_POINT ( 'NONE',  ( -19.37594187952227642, 20.00001632898912973, 230.3398175302317838 ) ) ;
#3270=DIRECTION ( 'NONE',  ( 1.000000000000000000, 0.000000000000000000, 0.000000000000000000 ) ) ;
#3302=CARTESIAN_POINT ( 'NONE',  ( -28.04325408110000240, 1.373251542630000035E-15, 230.2432540810000319 ) ) ;
#3339=CARTESIAN_POINT ( 'NONE',  ( 26.80000000000000071, -6.394884621839999216E-14, 230.6999999999999886 ) ) ;
#3382=CARTESIAN_POINT ( 'NONE',  ( 28.49999999970000175, 10.47094317839999889, 222.0000000000000000 ) ) ;
#3393=CARTESIAN_POINT ( 'NONE',  ( 19.32095615188756810, 19.99999286268905507, 230.3717215823191964 ) ) ;
#3400=CARTESIAN_POINT ( 'NONE',  ( -3.378474373710000034, -11.51459555979999827, 232.0000000000000000 ) ) ;
#3407=CARTESIAN_POINT ( 'NONE',  ( -0.2402207101440000103, -27.79943747540000132, 223.9202095490000204 ) ) ;
#3416=CARTESIAN_POINT ( 'NONE',  ( -23.79701075229709772, -14.37290030440138544, 225.9645151989870158 ) ) ;
#3454=CARTESIAN_POINT ( 'NONE',  ( 20.30405755279999980, 20.00000000000000000, 226.9999998930000231 ) ) ;
#3460=ADVANCED_FACE ( 'NONE', ( #7400 ), #19305, .F. ) ;
#3473=CARTESIAN_POINT ( 'NONE',  ( 28.49999999979999998, 4.812685681769999668, 229.0000000000000000 ) ) ;
#3477=ORIENTED_EDGE ( 'NONE', *, *, #3647, .T. ) ;
#3489=CARTESIAN_POINT ( 'NONE',  ( 24.91921101730000032, -13.83103916679999834, 223.9972514410000031 ) ) ;
#3490=CARTESIAN_POINT ( 'NONE',  ( -18.94276560960000211, 21.23709850699999890, 229.4982322489999831 ) ) ;
#3497=CARTESIAN_POINT ( 'NONE',  ( -15.84710441079999832, -21.98318857509999802, 230.6999999999999886 ) ) ;
#3532=CARTESIAN_POINT ( 'NONE',  ( 5.361384718760000112, -31.61859215249999977, 229.0000000000000000 ) ) ;
#3540=CARTESIAN_POINT ( 'NONE',  ( 25.26809617039999978, 12.77001320649999982, 222.0000000000000000 ) ) ;
#3553=CARTESIAN_POINT ( 'NONE',  ( 19.73226377590565050, 20.00031052610880877, 230.1021219667221089 ) ) ;
#3567=CARTESIAN_POINT ( 'NONE',  ( 28.45771199730000234, -1.659298224529999796E-14, 229.4982322489999831 ) ) ;
#3568=DIRECTION ( 'NONE',  ( 0.000000000000000000, 0.000000000000000000, 1.000000000000000000 ) ) ;
#3573=CARTESIAN_POINT ( 'NONE',  ( 0.5500237538654858538, -27.79507126796909944, 224.0359736129612145 ) ) ;
#3577=CARTESIAN_POINT ( 'NONE',  ( -20.04376857943106316, 19.99997512704260316, 229.7707830521836172 ) ) ;
#3614=ORIENTED_EDGE ( 'NONE', *, *, #26586, .F. ) ;
#3624=ADVANCED_FACE ( 'NONE', ( #6115 ), #16104, .F. ) ;
#3627=CARTESIAN_POINT ( 'NONE',  ( 24.61735023129999789, 13.67123892250000061, 230.5592437530000041 ) ) ;
#3641=CARTESIAN_POINT ( 'NONE',  ( 25.41516571979999739, -14.56554164990000011, 228.9999999990000106 ) ) ;
#3644=CARTESIAN_POINT ( 'NONE',  ( -26.80000000000000071, 4.518892556970000030, 230.6999999999999886 ) ) ;
#3647=EDGE_CURVE ( 'NONE', #11688, #27946, #24520, .T. ) ;
#3658=CARTESIAN_POINT ( 'NONE',  ( -25.11765555659999904, -13.46780168200000105, 225.6808342349999918 ) ) ;
#3672=CARTESIAN_POINT ( 'NONE',  ( -27.09307779339999911, 1.442401753589999799E-12, 229.9751247039999953 ) ) ;
#3673=B_SPLINE_CURVE_WITH_KNOTS ( 'NONE', 5,
 ( #12336, #12173, #17200, #19420, #26807, #24292, #21783, #552, #2740, #14863, #26352, #23997, #3039, #29010, #14552, #24454, #9662, #7607, #7310, #84, #2436, #19732, #12632, #19265 ),
 .UNSPECIFIED., .F., .F.,
 ( 6, 3, 3, 3, 3, 3, 3, 6 ),
 ( 0.000000000000000000, 11.88805610990000083, 23.77581053719999815, 35.66412908880000288, 47.55143447889999919, 59.43964105460000269, 71.32790799789999880, 81.23067401939999854 ),
 .UNSPECIFIED. ) ;
#3681=PRODUCT_DEFINITION_CONTEXT ( 'detailed design', #12597, 'design' ) ;
#3687=CARTESIAN_POINT ( 'NONE',  ( 24.46818569879999927, -13.19686604630000026, 224.2398747240000034 ) ) ;
#3696=CARTESIAN_POINT ( 'NONE',  ( 27.79999999990000248, 4.333901782529999025, 229.0000000000000000 ) ) ;
#3705=( LENGTH_UNIT ( ) NAMED_UNIT ( * ) SI_UNIT ( .MILLI., .METRE. ) );
#3710=CARTESIAN_POINT ( 'NONE',  ( 19.53679696397345822, 20.00007140946951623, 230.2446877367954130 ) ) ;
#3718=CARTESIAN_POINT ( 'NONE',  ( 28.49999999970000175, -7.466149220240000162, 229.0000000000000000 ) ) ;
#3724=CARTESIAN_POINT ( 'NONE',  ( -1.063084826889999945, -27.77996807399999923, 224.6898005070000011 ) ) ;
#3725=ORIENTED_EDGE ( 'NONE', *, *, #25276, .F. ) ;
#3732=( GEOMETRIC_REPRESENTATION_CONTEXT ( 3 ) GLOBAL_UNCERTAINTY_ASSIGNED_CONTEXT ( ( #30785 ) ) GLOBAL_UNIT_ASSIGNED_CONTEXT ( ( #28244, #6845, #25592 ) ) REPRESENTATION_CONTEXT ( 'NONE', 'WORKASPACE' ) );
#3736=CARTESIAN_POINT ( 'NONE',  ( 21.17691543559999801, 18.05241775060000009, 224.9999999359999947 ) ) ;
#3749=EDGE_CURVE ( 'NONE', #24996, #28749, #1616, .T. ) ;
#3752=EDGE_LOOP ( 'NONE', ( #7079, #285, #12350, #11072 ) ) ;
#3798=CARTESIAN_POINT ( 'NONE',  ( -0.8958568848479999680, -28.48628573779999940, 224.3198333100000070 ) ) ;
#3815=CARTESIAN_POINT ( 'NONE',  ( 24.69936741169999905, -14.21947533890000059, 223.9000014189999774 ) ) ;
#3816=CARTESIAN_POINT ( 'NONE',  ( -17.83931601680000156, 20.00000000000000000, 230.6999999999999886 ) ) ;
#3821=CARTESIAN_POINT ( 'NONE',  ( 12.06200471259999851, -24.13482272330000100, 230.6999999999999886 ) ) ;
#3828=ORIENTED_EDGE ( 'NONE', *, *, #3749, .F. ) ;
#3829=FACE_OUTER_BOUND ( 'NONE', #29994, .T. ) ;
#3840=CARTESIAN_POINT ( 'NONE',  ( -26.80000000000000071, -9.846360514330001479, 230.0000000000000000 ) ) ;
#3851=CARTESIAN_POINT ( 'NONE',  ( 24.68173674080000168, -14.25001227039999918, 223.9000014189999774 ) ) ;
#3862=CARTESIAN_POINT ( 'NONE',  ( 27.79999999990000248, 4.333901782529999025, 222.0000000000000000 ) ) ;
#3864=EDGE_CURVE ( 'NONE', #6498, #29484, #25242, .T. ) ;
#3904=ORIENTED_EDGE ( 'NONE', *, *, #22187, .F. ) ;
#3933=CARTESIAN_POINT ( 'NONE',  ( 0.8057459562559999844, -27.78864806999999715, 224.2403730839999980 ) ) ;
#3935=CARTESIAN_POINT ( 'NONE',  ( -27.98978497850000124, 6.821407819560000085, 222.0000000000000000 ) ) ;
#3950=ORIENTED_EDGE ( 'NONE', *, *, #2701, .F. ) ;
#3951=CARTESIAN_POINT ( 'NONE',  ( 22.51404573909999840, 18.05178744050000006, 229.4982322489999831 ) ) ;
#3952=B_SPLINE_CURVE_WITH_KNOTS ( 'NONE', 1,
 ( #12918, #19700 ),
 .UNSPECIFIED., .F., .F.,
 ( 2, 2 ),
 ( -2.556819966299999618E-06, 0.7000000000009999335 ),
 .UNSPECIFIED. ) ;
#3955=CARTESIAN_POINT ( 'NONE',  ( 6.818289962769999768, 16.85315611420000081, 230.6999999999999886 ) ) ;
#3969=CARTESIAN_POINT ( 'NONE',  ( 25.08428924680000094, -13.52916357279999993, 224.2398747240000034 ) ) ;
#3975=CARTESIAN_POINT ( 'NONE',  ( -19.80526803560000104, 19.50877411510000314, 228.5999999999999943 ) ) ;
#3988=ORIENTED_EDGE ( 'NONE', *, *, #4851, .T. ) ;
#3997=CARTESIAN_POINT ( 'NONE',  ( 27.09307779339999911, 1.385558334729999981E-12, 229.9751247039999953 ) ) ;
#4008=CARTESIAN_POINT ( 'NONE',  ( 24.73445225629999911, -14.15837998019999944, 223.9040346120000038 ) ) ;
#4018=EDGE_CURVE ( 'NONE', #11678, #29420, #20476, .T. ) ;
#4020=CARTESIAN_POINT ( 'NONE',  ( -28.50000000000000000, -5.472165930259999123E-14, 229.0000000000000000 ) ) ;
#4046=CARTESIAN_POINT ( 'NONE',  ( 27.56257419730000180, -5.215693983959999454E-14, 230.5592437530000041 ) ) ;
#4047=CARTESIAN_POINT ( 'NONE',  ( -1.809764279169999934, 12.20622105729999873, 232.6627643349999914 ) ) ;
#4051=CARTESIAN_POINT ( 'NONE',  ( 19.80538212960000166, 19.50875458629999670, 229.0000000010000178 ) ) ;
#4063=CARTESIAN_POINT ( 'NONE',  ( -24.09883371379999772, -15.21565466309999870, 224.8957841300000098 ) ) ;
#4064=EDGE_CURVE ( 'NONE', #10995, #18419, #18695, .T. ) ;
#4068=SHAPE_DEFINITION_REPRESENTATION ( #22894, #22833 ) ;
#4069=ORIENTED_EDGE ( 'NONE', *, *, #12913, .F. ) ;
#4076=CARTESIAN_POINT ( 'NONE',  ( 7.199615913319999727, -9.684780895279999413, 231.9999991140000191 ) ) ;
#4080=CARTESIAN_POINT ( 'NONE',  ( -27.29823224880000154, 7.105427357599999217E-15, 230.6577119970000069 ) ) ;
#4087=FACE_OUTER_BOUND ( 'NONE', #12239, .T. ) ;
#4105=EDGE_LOOP ( 'NONE', ( #7579, #7353, #19430 ) ) ;
#4116=ORIENTED_EDGE ( 'NONE', *, *, #29891, .T. ) ;
#4126=CARTESIAN_POINT ( 'NONE',  ( -23.66327188690000227, -14.59170227449999935, 225.7602679599999931 ) ) ;
#4132=CARTESIAN_POINT ( 'NONE',  ( 20.30405755279999980, 20.00000000000000000, 226.9999998930000231 ) ) ;
#4145=B_SPLINE_SURFACE_WITH_KNOTS ( 'NONE', 5, 1, ( 
 ( #25830, #4419 ),
 ( #20629, #4265 ),
 ( #21104, #1287 ),
 ( #30699, #18096 ),
 ( #27700, #6146 ),
 ( #3798, #7549 ),
 ( #20, #29102 ),
 ( #30853, #28643 ),
 ( #28952, #18892 ),
 ( #14024, #16990 ),
 ( #26744, #2063 ),
 ( #14175, #28786 ),
 ( #333, #26443 ),
 ( #21720, #26285 ),
 ( #23779, #19045 ) ),
 .UNSPECIFIED., .F., .F., .F.,
 ( 6, 3, 3, 3, 6 ),
 ( 2, 2 ),
 ( 0.000000000000000000, 0.5239015560140000138, 1.047803112029999983, 1.571704668039999975, 1.746338520049999898 ),
 ( -0.7000000000009999335, 2.556813327499999719E-06 ),
 .UNSPECIFIED. ) ;
#4146=ADVANCED_FACE ( 'NONE', ( #1873 ), #21571, .F. ) ;
#4153=CARTESIAN_POINT ( 'NONE',  ( 25.41516571979999739, -14.56554164990000011, 228.9999999990000106 ) ) ;
#4156=CARTESIAN_POINT ( 'NONE',  ( 25.64086108080000059, -11.13108427080000062, 222.0000000000000000 ) ) ;
#4172=CARTESIAN_POINT ( 'NONE',  ( 26.94142135619999934, -8.942955963489998358E-14, 230.0000000000000000 ) ) ;
#4199=CARTESIAN_POINT ( 'NONE',  ( 3.378474276019999945, 11.51459522689999915, 231.9999989789999972 ) ) ;
#4214=CARTESIAN_POINT ( 'NONE',  ( -23.50695179570000093, -14.84192241259999889, 225.0000014190000002 ) ) ;
#4231=B_SPLINE_CURVE_WITH_KNOTS ( 'NONE', 3,
 ( #14067, #26176, #16716, #9332, #63, #11855, #217, #14220, #2723, #23826, #21302, #21458 ),
 .UNSPECIFIED., .F., .F.,
 ( 4, 2, 2, 2, 2, 4 ),
 ( 0.000000000000000000, 0.1250000000000008049, 0.2500000000000016098, 0.5000000000000011102, 0.7500000000000005551, 1.000000000000000000 ),
 .UNSPECIFIED. ) ;
#4236=CARTESIAN_POINT ( 'NONE',  ( -14.02695468860000005, -28.16431168439999766, 229.7625741969999922 ) ) ;
#4265=CARTESIAN_POINT ( 'NONE',  ( -1.100001419170000050, -27.77850706310000106, 224.8959436220000043 ) ) ;
#4270=CARTESIAN_POINT ( 'NONE',  ( -25.20890834729999952, -13.29605215849999844, 225.3106485179999936 ) ) ;
#4290=CARTESIAN_POINT ( 'NONE',  ( 26.94142135619999934, 6.628004359539999533E-14, 230.0000000000000000 ) ) ;
#4295=CARTESIAN_POINT ( 'NONE',  ( -24.83650131330000121, 13.77747940670000126, 229.0000000000000000 ) ) ;
#4315=CARTESIAN_POINT ( 'NONE',  ( 26.28651405470000313, -11.41137627250000008, 222.0000000000000000 ) ) ;
#4327=CARTESIAN_POINT ( 'NONE',  ( 0.8738980057659999634, -27.78653623639999992, 225.6801530179999986 ) ) ;
#4330=ADVANCED_FACE ( 'NONE', ( #23242, #23409 ), #11738, .T. ) ;
#4342=CARTESIAN_POINT ( 'NONE',  ( -7.265484932596181444, 9.961462390592322080, 232.6627637660203050 ) ) ;
#4361=CARTESIAN_POINT ( 'NONE',  ( 3.378474373710000034, 11.51459555979999827, 232.0000000000000000 ) ) ;
#4362=CARTESIAN_POINT ( 'NONE',  ( -0.6521609806839999690, -27.79292263629999837, 225.9009104920000084 ) ) ;
#4363=CARTESIAN_POINT ( 'NONE',  ( 28.50000000000000000, 8.881784197000000993E-16, 222.0000000000000000 ) ) ;
#4370=CARTESIAN_POINT ( 'NONE',  ( -24.64674669169999888, -14.31123007319999907, 223.9013449489999914 ) ) ;
#4390=CARTESIAN_POINT ( 'NONE',  ( 19.90445648569999904, -20.03186682420000153, 230.6999999999999886 ) ) ;
#4391=VERTEX_POINT ( 'NONE', #24477 ) ;
#4396=CARTESIAN_POINT ( 'NONE',  ( 0.1059454459540000032, -28.50005195860000029, 223.9040507550000143 ) ) ;
#4403=CARTESIAN_POINT ( 'NONE',  ( 17.83930301670000418, 19.99998169580000251, 230.0000000000000000 ) ) ;
#4419=CARTESIAN_POINT ( 'NONE',  ( -1.100001419170000050, -27.77850706310000106, 225.0000014190000002 ) ) ;
#4421=CARTESIAN_POINT ( 'NONE',  ( -24.12724309970000292, -13.81083407110000039, 226.0959706989999916 ) ) ;
#4441=CARTESIAN_POINT ( 'NONE',  ( -24.66442003930000126, -14.28072947929999970, 226.1000014189999945 ) ) ;
#4451=ADVANCED_FACE ( 'NONE', ( #19289 ), #29900, .T. ) ;
#4461=B_SPLINE_CURVE_WITH_KNOTS ( 'NONE', 3,
 ( #19468, #7354, #28908, #7504, #17247, #24344, #4844, #14443, #5135, #12681, #2787, #26549 ),
 .UNSPECIFIED., .F., .F.,
 ( 4, 2, 2, 2, 2, 4 ),
 ( 0.000000000000000000, 0.2499999999999892308, 0.4999999999999784617, 0.6249999999999731326, 0.7499999999999676925, 1.000000000000000000 ),
 .UNSPECIFIED. ) ;
#4469=CARTESIAN_POINT ( 'NONE',  ( -26.17719569180000150, -11.91170824980000020, 222.0000000000000000 ) ) ;
#4506=ORIENTED_EDGE ( 'NONE', *, *, #2903, .T. ) ;
#4517=CARTESIAN_POINT ( 'NONE',  ( 19.29843289230000281, 19.63498672150000246, 229.6955567279999855 ) ) ;
#4518=CARTESIAN_POINT ( 'NONE',  ( -22.83911268609999823, 16.42879705509999866, 226.2000000000000171 ) ) ;
#4520=CARTESIAN_POINT ( 'NONE',  ( -0.2402207101440000103, -27.79943747540000132, 226.0797932899999978 ) ) ;
#4529=CARTESIAN_POINT ( 'NONE',  ( -24.09883371379999772, -15.21565466309999870, 225.0000014190000002 ) ) ;
#4545=CARTESIAN_POINT ( 'NONE',  ( -28.50000000000000000, 3.552713678799999608E-15, 229.2404163060000144 ) ) ;
#4572=CARTESIAN_POINT ( 'NONE',  ( 24.09856112909999837, -15.21545593799999985, 225.1041867410000350 ) ) ;
#4589=CARTESIAN_POINT ( 'NONE',  ( 26.80000000069999899, -3.214342854470000215E-14, 230.0000000000000000 ) ) ;
#4602=ORIENTED_EDGE ( 'NONE', *, *, #12558, .F. ) ;
#4607=CARTESIAN_POINT ( 'NONE',  ( 28.50000000000000000, -1.776356839399999804E-15, 229.0000000000000000 ) ) ;
#4611=EDGE_CURVE ( 'NONE', #1273, #13384, #22368, .T. ) ;
#4613=CARTESIAN_POINT ( 'NONE',  ( 10.97739439859999955, -26.47071190269999974, 222.0000000000000000 ) ) ;
#4615=CARTESIAN_POINT ( 'NONE',  ( 1.115119965759999943, -28.47834310740000063, 225.2081038119999903 ) ) ;
#4621=FACE_OUTER_BOUND ( 'NONE', #26466, .T. ) ;
#4626=CARTESIAN_POINT ( 'NONE',  ( -28.39963399990000070, 2.618402366230000222, 222.0000000000000000 ) ) ;
#4630=AXIS2_PLACEMENT_3D ( 'NONE', #14913, #7513, #12230 ) ;
#4654=CARTESIAN_POINT ( 'NONE',  ( 23.66291322330000213, -14.59162663150000050, 224.2398658380000143 ) ) ;
#4662=CARTESIAN_POINT ( 'NONE',  ( 17.83931934289999788, 20.00000000000000000, 229.9999934530000019 ) ) ;
#4670=CARTESIAN_POINT ( 'NONE',  ( 23.73489144358727998, -14.47434652104479191, 225.8865410910789251 ) ) ;
#4676=CIRCLE ( 'NONE', #21279, 1.700000000000000844 ) ;
#4693=CARTESIAN_POINT ( 'NONE',  ( 2.522786916459999862, -12.03261735549999933, 232.6627648150000027 ) ) ;
#4698=CARTESIAN_POINT ( 'NONE',  ( -28.35924375220000115, -10.41922902620000002, 229.7625741969999922 ) ) ;
#4721=FACE_OUTER_BOUND ( 'NONE', #17251, .T. ) ;
#4733=CARTESIAN_POINT ( 'NONE',  ( 23.52644129040000109, -14.81042608839999808, 225.3105549429999996 ) ) ;
#4740=CARTESIAN_POINT ( 'NONE',  ( -19.49313842129999941, 19.58644462790000063, 229.5590894759999969 ) ) ;
#4752=CARTESIAN_POINT ( 'NONE',  ( -17.83931601609999973, 20.00000000000000000, 230.0000000010000178 ) ) ;
#4760=VERTEX_POINT ( 'NONE', #30604 ) ;
#4799=CARTESIAN_POINT ( 'NONE',  ( 27.09307779339999911, -1.410781934549999973E-12, 229.9751247039999953 ) ) ;
#4802=EDGE_CURVE ( 'NONE', #21281, #29484, #13803, .T. ) ;
#4809=ADVANCED_FACE ( 'NONE', ( #4621 ), #25902, .T. ) ;
#4810=ORIENTED_EDGE ( 'NONE', *, *, #21781, .F. ) ;
#4825=EDGE_LOOP ( 'NONE', ( #14337, #9663, #15397, #16875 ) ) ;
#4829=CARTESIAN_POINT ( 'NONE',  ( -25.27355171200000328, 12.75978488059999805, 226.2000000000000171 ) ) ;
#4844=CARTESIAN_POINT ( 'NONE',  ( 24.22507564037507422, -15.01326821648306797, 224.3203909782756682 ) ) ;
#4851=EDGE_CURVE ( 'NONE', #14446, #1273, #780, .T. ) ;
#4855=CARTESIAN_POINT ( 'NONE',  ( 11.76719066729999774, -2.870640063430000222, 231.9999991140000191 ) ) ;
#4859=CARTESIAN_POINT ( 'NONE',  ( 27.56257419730000180, -5.329070518199999767E-14, 230.5592437530000041 ) ) ;
#4860=EDGE_LOOP ( 'NONE', ( #17286, #17172, #23952, #15060 ) ) ;
#4864=CARTESIAN_POINT ( 'NONE',  ( -1.100001419170000050, -27.77850706310000106, 225.0000014190000002 ) ) ;
#4913=CARTESIAN_POINT ( 'NONE',  ( -22.97554992469999746, 15.65135060219999907, 222.0000000000000000 ) ) ;
#4926=EDGE_CURVE ( 'NONE', #28330, #28642, #16417, .T. ) ;
#4927=CARTESIAN_POINT ( 'NONE',  ( 3.441895497200000431, 11.73074891959999988, 232.6627635220000059 ) ) ;
#4937=CARTESIAN_POINT ( 'NONE',  ( 23.55447120710000064, 16.04539730710000001, 222.0000000000000000 ) ) ;
#4939=TOROIDAL_SURFACE ( 'NONE', #2912, 18.16530045470000232, 1.699999999999999956 ) ;
#4963=CARTESIAN_POINT ( 'NONE',  ( 24.07552037900000030, -13.90000980950000020, 223.9000014189999774 ) ) ;
#4973=CARTESIAN_POINT ( 'NONE',  ( -1.870553977679999980, -12.14393525709999899, 232.6627643349999914 ) ) ;
#4977=CARTESIAN_POINT ( 'NONE',  ( 24.55235481438089096, -13.03932691102154351, 224.5041740165282533 ) ) ;
#4983=CARTESIAN_POINT ( 'NONE',  ( -1.871217229734078780, -11.95683611934309099, 232.0000002394077683 ) ) ;
#4988=CARTESIAN_POINT ( 'NONE',  ( -24.09302906149999757, -13.87041066189999938, 223.9000014189999774 ) ) ;
#5003=CARTESIAN_POINT ( 'NONE',  ( 12.04114732370000063, -0.8001383763589999809, 231.9999991140000191 ) ) ;
#5011=CARTESIAN_POINT ( 'NONE',  ( -0.8693959255619594373, -27.78669396130685953, 225.6773692761587142 ) ) ;
#5021=EDGE_CURVE ( 'NONE', #23376, #28017, #7382, .T. ) ;
#5120=CARTESIAN_POINT ( 'NONE',  ( -10.70571594490000145, -5.569299341639999845, 231.9999989789999972 ) ) ;
#5126=CARTESIAN_POINT ( 'NONE',  ( -21.20818545079999851, 16.99505982179999819, 230.0000000000000000 ) ) ;
#5134=CARTESIAN_POINT ( 'NONE',  ( -24.07583586439999834, -13.90018868249999962, 223.9000014189999774 ) ) ;
#5135=CARTESIAN_POINT ( 'NONE',  ( 24.16278207617288487, -15.11329356718511008, 224.5017226534712620 ) ) ;
#5147=CARTESIAN_POINT ( 'NONE',  ( 6.341353821860000295, 10.26877964679999877, 231.9999991140000191 ) ) ;
#5151=ORIENTED_EDGE ( 'NONE', *, *, #30602, .T. ) ;
#5176=ORIENTED_EDGE ( 'NONE', *, *, #23818, .F. ) ;
#5187=CARTESIAN_POINT ( 'NONE',  ( -21.70990266010000269, 18.50700188859999784, 225.0000000000000000 ) ) ;
#5224=CARTESIAN_POINT ( 'NONE',  ( -28.50000000000000000, -5.472165930259999123E-14, 229.0000000000000000 ) ) ;
#5300=ORIENTED_EDGE ( 'NONE', *, *, #13617, .F. ) ;
#5302=CARTESIAN_POINT ( 'NONE',  ( 25.11738521000000190, -13.46751580659999981, 225.6806823370000075 ) ) ;
#5329=CARTESIAN_POINT ( 'NONE',  ( -26.80000000000000071, 4.518892556989999143, 230.0000000000000000 ) ) ;
#5373=CARTESIAN_POINT ( 'NONE',  ( -1.419173393149999842E-06, -27.80022181310000207, 226.1000014189999945 ) ) ;
#5380=CARTESIAN_POINT ( 'NONE',  ( 27.44334449189999958, 9.611089166140001083, 229.4982322489999831 ) ) ;
#5381=CARTESIAN_POINT ( 'NONE',  ( -28.50000000000000000, 5.427757009279999762E-15, 222.0000000000000000 ) ) ;
#5384=B_SPLINE_CURVE_WITH_KNOTS ( 'NONE', 3,
 ( #1966, #23375, #28073, #6519, #1812, #30911, #25886, #18781, #30606, #28391, #11401, #6828, #28542, #16427, #11707, #27924, #9339, #6990 ),
 .UNSPECIFIED., .F., .F.,
 ( 4, 2, 2, 2, 2, 2, 2, 2, 4 ),
 ( 0.000000000000000000, 0.1249999999999999445, 0.2499999999999999445, 0.3749999999999999445, 0.5000000000000000000, 0.6250000000000000000, 0.7500000000000000000, 0.8749999999999998890, 1.000000000000000000 ),
 .UNSPECIFIED. ) ;
#5399=CARTESIAN_POINT ( 'NONE',  ( 18.32613298889999953, 20.54575842250000051, 229.7313256499999738 ) ) ;
#5432=AXIS2_PLACEMENT_3D ( 'NONE', #28018, #6614, #16217 ) ;
#5434=CARTESIAN_POINT ( 'NONE',  ( 23.83740787290000185, -14.30495753649999990, 223.9972528570000065 ) ) ;
#5449=EDGE_CURVE ( 'NONE', #27611, #30938, #23574, .T. ) ;
#5450=CARTESIAN_POINT ( 'NONE',  ( 24.68173674080000168, -14.25001227039999918, 226.1000014189999945 ) ) ;
#5476=CARTESIAN_POINT ( 'NONE',  ( -18.80296799075907543, 19.99998601668219678, 230.5746565848800742 ) ) ;
#5493=CARTESIAN_POINT ( 'NONE',  ( 24.05832192669999969, -13.92979812329999945, 226.1000014189999945 ) ) ;
#5501=CARTESIAN_POINT ( 'NONE',  ( -22.97554992469999746, 15.65135060219999907, 222.0000000000000000 ) ) ;
#5511=CARTESIAN_POINT ( 'NONE',  ( -26.80000000000000071, -8.704148513059999178E-14, 230.6999999999999886 ) ) ;
#5513=ADVANCED_FACE ( 'NONE', ( #7858 ), #27349, .F. ) ;
#5517=CARTESIAN_POINT ( 'NONE',  ( 0.8959394325020000327, -28.48619164239999790, 224.3198498209999912 ) ) ;
#5530=CARTESIAN_POINT ( 'NONE',  ( 28.49999999979999998, 4.812685681769999668, 229.2404163060000144 ) ) ;
#5531=CARTESIAN_POINT ( 'NONE',  ( 2.131628207279999844E-14, -1.704192342799999938E-14, 230.7531949689999919 ) ) ;
#5534=CARTESIAN_POINT ( 'NONE',  ( -19.80526803560000104, 19.50877411510000314, 229.0000000000000000 ) ) ;
#5542=CARTESIAN_POINT ( 'NONE',  ( -1.127665019380140299, -28.47796022461074728, 224.8525238069234717 ) ) ;
#5545=CARTESIAN_POINT ( 'NONE',  ( 27.72013230379999627, 7.265883530940000057, 222.0000000000000000 ) ) ;
#5550=CARTESIAN_POINT ( 'NONE',  ( 27.79999999980000069, 4.694479351150000035, 229.0000000000000000 ) ) ;
#5569=CARTESIAN_POINT ( 'NONE',  ( -27.71720220699999970, -10.18334195910000162, 229.4485730569999760 ) ) ;
#5576=EDGE_LOOP ( 'NONE', ( #3828, #23182, #2175, #1277 ) ) ;
#5579=ADVANCED_FACE ( 'NONE', ( #11596 ), #12014, .F. ) ;
#5580=CARTESIAN_POINT ( 'NONE',  ( 17.83930301670000418, 19.99998169580000251, 230.0000000000000000 ) ) ;
#5585=CARTESIAN_POINT ( 'NONE',  ( 23.62697774660000150, -14.64965012220000062, 224.3193082299999901 ) ) ;
#5590=FILL_AREA_STYLE_COLOUR ( '', #25868 ) ;
#5599=DIRECTION ( 'NONE',  ( 0.000000000000000000, 0.000000000000000000, -1.000000000000000000 ) ) ;
#5601=ADVANCED_FACE ( 'NONE', ( #23718 ), #19043, .F. ) ;
#5626=CARTESIAN_POINT ( 'NONE',  ( -24.00375951252449269, -14.02501865426384775, 226.1000014189999376 ) ) ;
#5631=CARTESIAN_POINT ( 'NONE',  ( -18.62251649170634238, 19.99999711498608690, 230.6160300935700036 ) ) ;
#5647=VERTEX_POINT ( 'NONE', #10776 ) ;
#5665=CARTESIAN_POINT ( 'NONE',  ( -24.60699597083884171, -12.93667822868543738, 225.1470444808221885 ) ) ;
#5671=ORIENTED_EDGE ( 'NONE', *, *, #1024, .T. ) ;
#5683=CARTESIAN_POINT ( 'NONE',  ( 27.29823224869999976, 4.609747771270000349, 230.6577119970000069 ) ) ;
#5697=CARTESIAN_POINT ( 'NONE',  ( 27.79999999980000069, -7.282770092329999834, 229.0000000000000000 ) ) ;
#5700=CARTESIAN_POINT ( 'NONE',  ( -25.84755624059999946, 9.037785233809998431, 230.6999999999999886 ) ) ;
#5713=ADVANCED_FACE ( 'NONE', ( #17682, #27298, #5741, #22592 ), #30784, .F. ) ;
#5715=ORIENTED_EDGE ( 'NONE', *, *, #17830, .T. ) ;
#5729=CARTESIAN_POINT ( 'NONE',  ( -27.79999999999999716, -2.375185619369999834, 222.0000000000000000 ) ) ;
#5741=FACE_BOUND ( 'NONE', #21997, .T. ) ;
#5749=CARTESIAN_POINT ( 'NONE',  ( -5.361385120510000490, 31.61859227569999931, 222.0000000000000000 ) ) ;
#5777=ADVANCED_FACE ( 'NONE', ( #2119 ), #9164, .F. ) ;
#5787=B_SPLINE_CURVE_WITH_KNOTS ( 'NONE', 1,
 ( #22291, #27461 ),
 .UNSPECIFIED., .F., .F.,
 ( 2, 2 ),
 ( -2.557517344899999924E-06, 0.7000000000009999335 ),
 .UNSPECIFIED. ) ;
#5790=CARTESIAN_POINT ( 'NONE',  ( -18.57884138570541310, 20.00001926002121166, 230.6254606444483386 ) ) ;
#5809=CARTESIAN_POINT ( 'NONE',  ( -22.36167894509999954, 17.71395549689999882, 224.0000000000000000 ) ) ;
#5820=CARTESIAN_POINT ( 'NONE',  ( 0.2402089773019999985, -27.79941220630000132, 226.0797949779999954 ) ) ;
#5832=VERTEX_POINT ( 'NONE', #21627 ) ;
#5849=CARTESIAN_POINT ( 'NONE',  ( 3.550686847520000117E-05, -28.50022181210000127, 223.9000014189999774 ) ) ;
#5851=CARTESIAN_POINT ( 'NONE',  ( 25.11738521000000190, -13.46751580659999981, 224.3193205009999929 ) ) ;
#5852=CARTESIAN_POINT ( 'NONE',  ( -27.29823224869999976, 4.602902183869999497, 230.6577119970000069 ) ) ;
#5854=CARTESIAN_POINT ( 'NONE',  ( 27.79999999980000069, -7.282770092339999835, 222.0000000000000000 ) ) ;
#5855=CARTESIAN_POINT ( 'NONE',  ( -25.89944370639999960, -7.563310173900000599, 230.6999999999999886 ) ) ;
#5873=CARTESIAN_POINT ( 'NONE',  ( -27.79999999970000246, -10.21376199200000201, 229.1414213560000235 ) ) ;
#5888=CARTESIAN_POINT ( 'NONE',  ( -28.50000000000000000, 4.144832625269998950E-15, 229.0000000000000000 ) ) ;
#5893=CARTESIAN_POINT ( 'NONE',  ( 27.79999999999999716, 2.355804440410000085E-11, 229.0000000000000000 ) ) ;
#5897=CARTESIAN_POINT ( 'NONE',  ( -21.16705332929999983, 21.30254446269999846, 222.0000000000000000 ) ) ;
#5909=CARTESIAN_POINT ( 'NONE',  ( 18.59546134273585594, 19.99999462727945243, 230.6223120414987875 ) ) ;
#5930=CARTESIAN_POINT ( 'NONE',  ( 19.80538173989999962, 19.50875420239999869, 227.7999999360000061 ) ) ;
#5932=CARTESIAN_POINT ( 'NONE',  ( -23.93349116070633542, -14.14448167692421876, 226.0729041749974044 ) ) ;
#5938=CARTESIAN_POINT ( 'NONE',  ( -19.88589761007506596, 20.00023699978923730, 229.9605059376604856 ) ) ;
#5956=AXIS2_PLACEMENT_3D ( 'NONE', #7784, #9688, #19291 ) ;
#5993=CARTESIAN_POINT ( 'NONE',  ( 26.58011360040000071, 9.308772197099999701, 230.5592437530000041 ) ) ;
#6009=CARTESIAN_POINT ( 'NONE',  ( -22.55348085480000364, 18.07310466269999694, 229.2404163060000144 ) ) ;
#6014=CARTESIAN_POINT ( 'NONE',  ( -27.79999999970000246, -10.21376199200000201, 229.0000000000000000 ) ) ;
#6015=CARTESIAN_POINT ( 'NONE',  ( 14.81012440339999969, 10.71727884689999932, 230.6999999999999886 ) ) ;
#6023=CARTESIAN_POINT ( 'NONE',  ( 20.30405755279999980, 20.00000000000000000, 226.9999998930000231 ) ) ;
#6033=CARTESIAN_POINT ( 'NONE',  ( -26.80000000000000071, 3.552713678799999608E-15, 230.0000000000000000 ) ) ;
#6046=B_SPLINE_CURVE_WITH_KNOTS ( 'NONE', 5,
 ( #12948, #18282, #1143, #10737, #1002, #20652, #20336, #17957, #8058, #15459, #22557, #8362, #30250, #29934, #27725, #20183, #8680, #6015, #27889, #6333, #29775, #1618, #15930, #15613 ),
 .UNSPECIFIED., .F., .F.,
 ( 6, 3, 3, 3, 3, 3, 3, 6 ),
 ( 0.000000000000000000, 11.88805619960000115, 23.77581072610000135, 35.66412938380000242, 47.55143485110000512, 59.43964151330000334, 71.32790854499999966, 76.96280491019999204 ),
 .UNSPECIFIED. ) ;
#6049=CARTESIAN_POINT ( 'NONE',  ( -23.69119896560000171, -20.94188573509999785, 229.0000000000000000 ) ) ;
#6059=CARTESIAN_POINT ( 'NONE',  ( 27.79999999999999716, -2.355749216199999846E-11, 224.8000000000000114 ) ) ;
#6069=CARTESIAN_POINT ( 'NONE',  ( 20.30405755288911251, 20.00000000000103384, 229.0659093385340839 ) ) ;
#6114=CARTESIAN_POINT ( 'NONE',  ( 20.64716981389999972, -20.77933506589999979, 222.0000000000000000 ) ) ;
#6115=FACE_OUTER_BOUND ( 'NONE', #9634, .T. ) ;
#6132=CARTESIAN_POINT ( 'NONE',  ( 0.1059454459540000032, -28.50005195860000029, 223.9040507550000143 ) ) ;
#6146=CARTESIAN_POINT ( 'NONE',  ( -0.9902521520970002378, -27.78273347009999839, 224.4935097720000101 ) ) ;
#6149=CARTESIAN_POINT ( 'NONE',  ( -24.30742244210000180, -13.49161940289999961, 226.0028092389999870 ) ) ;
#6161=CARTESIAN_POINT ( 'NONE',  ( -17.83931601680000156, 20.00000000000000000, 230.7000111870000012 ) ) ;
#6163=ADVANCED_FACE ( 'NONE', ( #9147 ), #6654, .T. ) ;
#6164=CARTESIAN_POINT ( 'NONE',  ( -28.04325408099999706, 4.728524333599999352, 230.2432540810000319 ) ) ;
#6166=CARTESIAN_POINT ( 'NONE',  ( -24.22223838309999877, -15.01863363589999878, 225.6808321819999890 ) ) ;
#6170=CARTESIAN_POINT ( 'NONE',  ( -11.38367146589999912, -24.46198237100000128, 230.6999999999999886 ) ) ;
#6186=CARTESIAN_POINT ( 'NONE',  ( 5.114250173089999407, 17.43050732989999929, 231.6999999999999886 ) ) ;
#6194=CARTESIAN_POINT ( 'NONE',  ( -13.32567267019999946, -26.75623947960000137, 230.0000000000000000 ) ) ;
#6195=CARTESIAN_POINT ( 'NONE',  ( -19.80526803560000104, 19.50877411510000314, 227.0000000000000000 ) ) ;
#6203=CARTESIAN_POINT ( 'NONE',  ( 19.06862361850000198, 19.69237242210000005, 229.7996270940000159 ) ) ;
#6205=CARTESIAN_POINT ( 'NONE',  ( 24.50046877880000196, -13.13673243530000079, 224.3193205009999929 ) ) ;
#6215=FACE_OUTER_BOUND ( 'NONE', #26942, .T. ) ;
#6223=CARTESIAN_POINT ( 'NONE',  ( -8.915308721984681384, -8.516764330229598556, 232.6627637660201628 ) ) ;
#6227=CARTESIAN_POINT ( 'NONE',  ( 18.28303642507142968, 20.00000852599190537, 230.6738034682653904 ) ) ;
#6231=CARTESIAN_POINT ( 'NONE',  ( -19.29867024690000221, 19.63492390480000083, 229.6953880050000123 ) ) ;
#6235=CARTESIAN_POINT ( 'NONE',  ( 24.66410523950000311, -14.28055064019999953, 226.1000014189999945 ) ) ;
#6252=CARTESIAN_POINT ( 'NONE',  ( -24.09883371379999772, -15.21565466309999870, 225.1042187089999800 ) ) ;
#6259=CARTESIAN_POINT ( 'NONE',  ( -20.30396346370000060, 20.00000000000000000, 229.0000000000000000 ) ) ;
#6281=CARTESIAN_POINT ( 'NONE',  ( -1.419173393149999842E-06, -27.80022181310000207, 226.1000014189999945 ) ) ;
#6289=EDGE_CURVE ( 'NONE', #10995, #6418, #23900, .T. ) ;
#6291=CARTESIAN_POINT ( 'NONE',  ( 0.1033071333860000052, -27.80005613160000166, 223.9040507550000143 ) ) ;
#6293=CARTESIAN_POINT ( 'NONE',  ( -28.50000000000000000, 1.776356839399999922E-14, 222.0000000000000000 ) ) ;
#6305=CARTESIAN_POINT ( 'NONE',  ( -25.17394274020000111, -13.36230406159999973, 224.4928762930000232 ) ) ;
#6313=CARTESIAN_POINT ( 'NONE',  ( 21.39276574850000046, 17.15274395180000155, 230.6999999999999886 ) ) ;
#6315=CARTESIAN_POINT ( 'NONE',  ( -19.80526744909999692, 19.50877353739999975, 229.0000000010000178 ) ) ;
#6316=CARTESIAN_POINT ( 'NONE',  ( -24.07583586439999834, -13.90018868249999962, 226.1000014189999945 ) ) ;
#6328=CARTESIAN_POINT ( 'NONE',  ( 25.17364887440000132, -13.36205984489999921, 224.4930265309999982 ) ) ;
#6332=FACE_BOUND ( 'NONE', #17815, .T. ) ;
#6333=CARTESIAN_POINT ( 'NONE',  ( 12.00334263380000088, 13.78333882559999957, 230.6999999999999886 ) ) ;
#6392=VERTEX_POINT ( 'NONE', #19496 ) ;
#6402=CARTESIAN_POINT ( 'NONE',  ( 17.99586598600000187, 19.96083381589999917, 229.9999934530000019 ) ) ;
#6414=CARTESIAN_POINT ( 'NONE',  ( -20.30396346370000060, 20.00000000000000000, 227.8000000000000114 ) ) ;
#6418=VERTEX_POINT ( 'NONE', #2266 ) ;
#6423=VECTOR ( 'NONE', #12768, 1000.000000000000114 ) ;
#6431=CARTESIAN_POINT ( 'NONE',  ( -5.509622826249999328, -10.91334849979999966, 232.6627648150000027 ) ) ;
#6454=CARTESIAN_POINT ( 'NONE',  ( -25.00949650980000172, -13.66806287920000074, 224.0985996330000205 ) ) ;
#6464=CARTESIAN_POINT ( 'NONE',  ( -26.95773188389999930, 8.656139546040000354, 229.0000000000000000 ) ) ;
#6469=AXIS2_PLACEMENT_3D ( 'NONE', #19802, #29388, #24674 ) ;
#6481=CARTESIAN_POINT ( 'NONE',  ( -23.50695179570000093, -14.84192241259999889, 225.1042187089999800 ) ) ;
#6498=VERTEX_POINT ( 'NONE', #12316 ) ;
#6508=CARTESIAN_POINT ( 'NONE',  ( -13.75032424529999986, -27.60893268180000248, 229.0000000050000040 ) ) ;
#6510=CARTESIAN_POINT ( 'NONE',  ( 26.49877067279999920, -8.898240373709999318, 222.0000000000000000 ) ) ;
#6519=CARTESIAN_POINT ( 'NONE',  ( 8.915309161273842875, 8.516764744512210328, 232.6627635626987853 ) ) ;
#6521=CARTESIAN_POINT ( 'NONE',  ( 24.80399018339999628, -14.03663607480000053, 223.9201473980000117 ) ) ;
#6523=CARTESIAN_POINT ( 'NONE',  ( -28.50000000000000000, 0.8733855473370000233, 222.0000000000000000 ) ) ;
#6538=CARTESIAN_POINT ( 'NONE',  ( -8.516764330228012270, 8.915308721986194840, 232.6627637660202765 ) ) ;
#6540=ORIENTED_EDGE ( 'NONE', *, *, #16660, .T. ) ;
#6545=CARTESIAN_POINT ( 'NONE',  ( 19.80538212960000166, 19.50875458629999670, 229.0000000010000178 ) ) ;
#6556=CARTESIAN_POINT ( 'NONE',  ( 18.41899666859999840, 20.00000949010000184, 230.6632774530000063 ) ) ;
#6559=CARTESIAN_POINT ( 'NONE',  ( -1.015151870880000029, -28.48229306780000059, 225.5064930660000186 ) ) ;
#6571=CARTESIAN_POINT ( 'NONE',  ( -23.95524095760000094, -14.10746636989999914, 223.9201349020000009 ) ) ;
#6590=CARTESIAN_POINT ( 'NONE',  ( 26.80000000000000071, -7.020799968500000432, 230.6999999999999886 ) ) ;
#6597=CARTESIAN_POINT ( 'NONE',  ( 0.9902601295740001142, -27.78262976010000074, 224.4935313260000100 ) ) ;
#6614=DIRECTION ( 'NONE',  ( 0.000000000000000000, 0.000000000000000000, -1.000000000000000000 ) ) ;
#6626=CARTESIAN_POINT ( 'NONE',  ( -18.15350094950000326, 19.92137095469999863, 229.9929676959999938 ) ) ;
#6654=B_SPLINE_SURFACE_WITH_KNOTS ( 'NONE', 5, 1, ( 
 ( #8996, #18748 ),
 ( #28037, #6481 ),
 ( #11366, #21273 ),
 ( #28351, #30569 ),
 ( #23645, #6796 ),
 ( #6166, #18278 ),
 ( #25850, #4126 ),
 ( #13569, #11674 ),
 ( #20649, #9307 ),
 ( #23333, #11205 ),
 ( #30877, #11057 ),
 ( #1615, #25999 ),
 ( #28193, #13722 ),
 ( #4441, #27722 ),
 ( #25381, #23492 ) ),
 .UNSPECIFIED., .F., .F., .F.,
 ( 6, 3, 3, 3, 6 ),
 ( 2, 2 ),
 ( 0.000000000000000000, 0.5239055193870000293, 1.047811038780000148, 1.571716558160000110, 1.746351731290000098 ),
 ( -0.7000000000009999335, 2.557291473029999731E-06 ),
 .UNSPECIFIED. ) ;
#6662=CARTESIAN_POINT ( 'NONE',  ( 20.95194113719999862, -19.55023117750000239, 222.0000000000000000 ) ) ;
#6674=CARTESIAN_POINT ( 'NONE',  ( -27.76736547790000031, 1.703869260230000071, 222.0000000000000000 ) ) ;
#6680=ORIENTED_EDGE ( 'NONE', *, *, #8815, .T. ) ;
#6710=CARTESIAN_POINT ( 'NONE',  ( -1.776417072969999733, 11.98130592599999922, 231.9999989789999972 ) ) ;
#6714=FACE_OUTER_BOUND ( 'NONE', #22956, .T. ) ;
#6716=CARTESIAN_POINT ( 'NONE',  ( 1.070950144331349163, -27.77958776724596746, 224.7107472884561048 ) ) ;
#6723=CARTESIAN_POINT ( 'NONE',  ( -24.62906106470000012, -14.34164290000000008, 223.9040321109999923 ) ) ;
#6740=CARTESIAN_POINT ( 'NONE',  ( -4.962952493270000431, -10.92748134360000023, 231.9999991140000191 ) ) ;
#6745=CARTESIAN_POINT ( 'NONE',  ( 5.334905827900000119, -31.46243374959999883, 229.7625741969999922 ) ) ;
#6753=CARTESIAN_POINT ( 'NONE',  ( -24.09302906149999757, -13.87041066189999938, 223.9000014189999774 ) ) ;
#6759=DIRECTION ( 'NONE',  ( 0.4353787270609797422, 0.9002473904559573636, 0.000000000000000000 ) ) ;
#6762=EDGE_CURVE ( 'NONE', #17135, #28330, #22706, .T. ) ;
#6772=EDGE_CURVE ( 'NONE', #13384, #18572, #26827, .T. ) ;
#6776=CARTESIAN_POINT ( 'NONE',  ( 18.17096580360000146, 20.37181511329999850, 230.6577119970000069 ) ) ;
#6777=CIRCLE ( 'NONE', #28390, 1.700000000000000178 ) ;
#6780=CARTESIAN_POINT ( 'NONE',  ( -25.00949650969999993, -13.66806287920000074, 225.9014032059999977 ) ) ;
#6787=CARTESIAN_POINT ( 'NONE',  ( -18.80718603000000044, 20.00000136549999752, 230.5856263059999947 ) ) ;
#6795=CARTESIAN_POINT ( 'NONE',  ( -27.30231674030000022, 6.653883447060000123, 222.0000000000000000 ) ) ;
#6796=CARTESIAN_POINT ( 'NONE',  ( -23.56565371579999990, -14.74874063789999923, 225.5071239680000303 ) ) ;
#6800=ADVANCED_FACE ( 'NONE', ( #30856 ), #1888, .F. ) ;
#6803=CARTESIAN_POINT ( 'NONE',  ( -27.77512470410000134, 4.683313577610000777, 229.2930777930000090 ) ) ;
#6810=CARTESIAN_POINT ( 'NONE',  ( -22.03726251081861065, 17.02871019621900217, 223.6666666666666572 ) ) ;
#6820=CARTESIAN_POINT ( 'NONE',  ( 5.125960221229999725, -30.23021873609999943, 229.9172029869999960 ) ) ;
#6822=CARTESIAN_POINT ( 'NONE',  ( -3.423281690950000122, -28.45174682580000081, 222.0000000000000000 ) ) ;
#6828=CARTESIAN_POINT ( 'NONE',  ( 8.516764494467457425, -8.915308899531273923, 232.6627636846916403 ) ) ;
#6833=CARTESIAN_POINT ( 'NONE',  ( 1.127732790480000080, -28.47784299079999926, 225.0000014190000002 ) ) ;
#6845=( NAMED_UNIT ( * ) PLANE_ANGLE_UNIT ( ) SI_UNIT ( $, .RADIAN. ) );
#6861=CARTESIAN_POINT ( 'NONE',  ( 24.48837202150000181, -14.58033361329999877, 226.0424736289999714 ) ) ;
#6863=CARTESIAN_POINT ( 'NONE',  ( 19.56378028550000181, 19.56885116670000357, 229.4995147189999898 ) ) ;
#6871=CARTESIAN_POINT ( 'NONE',  ( -26.94142135619999934, -1.740902259209999758E-13, 230.0000000000000000 ) ) ;
#6875=CARTESIAN_POINT ( 'NONE',  ( -24.15901410609999900, -15.12012600329999934, 224.4928788709999878 ) ) ;
#6894=CARTESIAN_POINT ( 'NONE',  ( 5.275462242469999730, -31.11186713239999690, 230.2432540810000319 ) ) ;
#6903=CARTESIAN_POINT ( 'NONE',  ( 0.2462945485190000117, -28.49939181899999951, 223.9202078600000050 ) ) ;
#6904=CARTESIAN_POINT ( 'NONE',  ( 22.41293933140000050, 16.47772227400000489, 222.9999999789999947 ) ) ;
#6907=AXIS2_PLACEMENT_3D ( 'NONE', #16184, #21074, #16341 ) ;
#6966=CARTESIAN_POINT ( 'NONE',  ( 22.36196472700000015, 17.71394650440000262, 223.9999999570000000 ) ) ;
#6979=VERTEX_POINT ( 'NONE', #12272 ) ;
#6982=CARTESIAN_POINT ( 'NONE',  ( 14.99213822049999933, -23.71131899119999886, 222.0000000000000000 ) ) ;
#6987=ADVANCED_FACE ( 'NONE', ( #11814 ), #16199, .F. ) ;
#6990=CARTESIAN_POINT ( 'NONE',  ( -3.441895295100000141, -11.73074823080000151, 232.6627637660000119 ) ) ;
#6994=CARTESIAN_POINT ( 'NONE',  ( -26.28649255380000227, 11.41136534319999996, 222.0000000000000000 ) ) ;
#7027=CARTESIAN_POINT ( 'NONE',  ( 24.68173674080000168, -14.25001227039999918, 226.1000014189999945 ) ) ;
#7028=CARTESIAN_POINT ( 'NONE',  ( 18.03079990150000000, 20.00000068800000008, 230.7000122960000112 ) ) ;
#7029=CARTESIAN_POINT ( 'NONE',  ( -19.80526803560000104, 19.50877411520000138, 222.0000000000000000 ) ) ;
#7031=CARTESIAN_POINT ( 'NONE',  ( -0.07056952541309999272, -28.50017087330000010, 226.0986539140000104 ) ) ;
#7034=CARTESIAN_POINT ( 'NONE',  ( 24.07552309629999954, -13.90001137829999855, 226.1000014189999945 ) ) ;
#7036=CARTESIAN_POINT ( 'NONE',  ( 12.09920926763414073, -0.2766206855562842737, 232.0000002394077967 ) ) ;
#7037=CARTESIAN_POINT ( 'NONE',  ( -27.09307779339999911, -1.459363161060000088E-12, 229.9751247039999953 ) ) ;
#7042=CARTESIAN_POINT ( 'NONE',  ( -24.68204616399999907, -14.25020164319999871, 223.9000014189999774 ) ) ;
#7050=CARTESIAN_POINT ( 'NONE',  ( 25.90432029460000152, 13.09158661030000026, 229.0000000000000000 ) ) ;
#7053=CARTESIAN_POINT ( 'NONE',  ( -22.36167894509999954, 17.71395549689999882, 224.0000000000000000 ) ) ;
#7057=CARTESIAN_POINT ( 'NONE',  ( -28.04325408110000240, 1.065814103639999922E-14, 230.2432540810000319 ) ) ;
#7065=CARTESIAN_POINT ( 'NONE',  ( 22.97596755210000197, 15.65128466780000061, 222.0000000000000000 ) ) ;
#7079=ORIENTED_EDGE ( 'NONE', *, *, #30030, .F. ) ;
#7090=CARTESIAN_POINT ( 'NONE',  ( 23.51325844009999955, -14.83130343779999905, 225.2083717279999746 ) ) ;
#7092=CARTESIAN_POINT ( 'NONE',  ( 5.023648568059999597, 17.12171681569999748, 230.7531949689999919 ) ) ;
#7097=CARTESIAN_POINT ( 'NONE',  ( -19.56389390649999882, 19.56881929660000097, 229.4993219170000032 ) ) ;
#7111=DIRECTION ( 'NONE',  ( 0.000000000000000000, 0.000000000000000000, -1.000000000000000000 ) ) ;
#7121=EDGE_CURVE ( 'NONE', #19036, #2003, #16049, .T. ) ;
#7135=CARTESIAN_POINT ( 'NONE',  ( 3.550686850769999806E-05, -28.50022181210000127, 226.1000014189999945 ) ) ;
#7140=DIRECTION ( 'NONE',  ( 0.000000000000000000, 0.000000000000000000, 1.000000000000000000 ) ) ;
#7159=ORIENTED_EDGE ( 'NONE', *, *, #4926, .F. ) ;
#7172=CARTESIAN_POINT ( 'NONE',  ( 23.62697774660000150, -14.64965012220000062, 224.3193082299999901 ) ) ;
#7174=DIRECTION ( 'NONE',  ( 0.000000000000000000, 0.000000000000000000, -1.000000000000000000 ) ) ;
#7179=CARTESIAN_POINT ( 'NONE',  ( -0.8513360036590000846, -12.01011570999999911, 231.9999989789999972 ) ) ;
#7181=CARTESIAN_POINT ( 'NONE',  ( -22.83911268609999823, 16.42879705520000044, 222.0000000000000000 ) ) ;
#7187=CARTESIAN_POINT ( 'NONE',  ( 23.93355402185607872, -14.14369205957050468, 226.0731811994463669 ) ) ;
#7215=CARTESIAN_POINT ( 'NONE',  ( 25.92643298289999976, -14.85855223419999938, 229.7625741969999922 ) ) ;
#7219=CARTESIAN_POINT ( 'NONE',  ( -27.79999999999999716, -2.360778239559999931E-11, 229.0000000000000000 ) ) ;
#7240=VERTEX_POINT ( 'NONE', #16758 ) ;
#7271=ORIENTED_EDGE ( 'NONE', *, *, #22721, .T. ) ;
#7302=CARTESIAN_POINT ( 'NONE',  ( 25.98552618960000160, 10.26029398309999863, 222.0000000000000000 ) ) ;
#7310=CARTESIAN_POINT ( 'NONE',  ( -13.76031144620000113, -12.03544455119999945, 230.6999999999999886 ) ) ;
#7320=CARTESIAN_POINT ( 'NONE',  ( 21.88912777999999903, 15.65358089960000321, 230.6999999999999886 ) ) ;
#7330=CARTESIAN_POINT ( 'NONE',  ( 23.83740787290000185, -14.30495753649999990, 223.9972528570000065 ) ) ;
#7353=ORIENTED_EDGE ( 'NONE', *, *, #6772, .F. ) ;
#7354=CARTESIAN_POINT ( 'NONE',  ( 24.60810180234884825, -14.37755052939759715, 223.9000014190000627 ) ) ;
#7356=ORIENTED_EDGE ( 'NONE', *, *, #9844, .F. ) ;
#7369=ORIENTED_EDGE ( 'NONE', *, *, #20595, .T. ) ;
#7373=CARTESIAN_POINT ( 'NONE',  ( -27.79999999999999716, -2.354383354940000152E-11, 222.0000000000000000 ) ) ;
#7382=B_SPLINE_CURVE_WITH_KNOTS ( 'NONE', 3,
 ( #5849, #24747, #7897, #17503, #17949, #692, #10279, #543, #24907, #27259, #5542, #22694 ),
 .UNSPECIFIED., .F., .F.,
 ( 4, 2, 2, 2, 2, 4 ),
 ( 0.000000000000000000, 0.2500000000000267009, 0.5000000000000534017, 0.6250000000000505151, 0.7500000000000476286, 1.000000000000000000 ),
 .UNSPECIFIED. ) ;
#7400=FACE_OUTER_BOUND ( 'NONE', #8418, .T. ) ;
#7424=CARTESIAN_POINT ( 'NONE',  ( 24.68173674080000168, -14.25001227039999918, 226.1000014189999945 ) ) ;
#7458=CARTESIAN_POINT ( 'NONE',  ( 27.79999999999999716, 2.355804440410000085E-11, 229.0000000000000000 ) ) ;
#7463=ORIENTED_EDGE ( 'NONE', *, *, #17830, .F. ) ;
#7487=CARTESIAN_POINT ( 'NONE',  ( -6.652733932600000344, -10.33873597240000031, 232.6627643349999914 ) ) ;
#7488=CARTESIAN_POINT ( 'NONE',  ( -27.79999999999999716, -2.356928386389999887E-11, 224.8000000000000114 ) ) ;
#7489=CARTESIAN_POINT ( 'NONE',  ( 23.56533302370000271, -14.74861233630000079, 224.4930104139999969 ) ) ;
#7497=CARTESIAN_POINT ( 'NONE',  ( 8.751033282710258376, 8.359832557568292799, 232.0000002394078251 ) ) ;
#7504=CARTESIAN_POINT ( 'NONE',  ( 24.39644993330914247, -14.73373303253482369, 224.0345656044051168 ) ) ;
#7513=DIRECTION ( 'NONE',  ( 0.000000000000000000, 0.000000000000000000, -1.000000000000000000 ) ) ;
#7535=CARTESIAN_POINT ( 'NONE',  ( -24.07583586439999834, -13.90018868249999962, 223.9000014189999774 ) ) ;
#7536=CARTESIAN_POINT ( 'NONE',  ( -24.81427761910000029, 13.76515143070000136, 229.2930779689999952 ) ) ;
#7548=ORIENTED_EDGE ( 'NONE', *, *, #532, .T. ) ;
#7549=CARTESIAN_POINT ( 'NONE',  ( -0.8738876050350000702, -27.78662806160000187, 224.3198333100000070 ) ) ;
#7550=EDGE_LOOP ( 'NONE', ( #8499, #27577, #18166, #10679 ) ) ;
#7551=CARTESIAN_POINT ( 'NONE',  ( 24.09856112909999837, -15.21545593799999985, 225.0000014190000002 ) ) ;
#7579=ORIENTED_EDGE ( 'NONE', *, *, #24242, .F. ) ;
#7587=ADVANCED_FACE ( 'NONE', ( #11084 ), #23511, .F. ) ;
#7601=CARTESIAN_POINT ( 'NONE',  ( -17.83931601609999973, 20.00000000000000000, 230.0000000010000178 ) ) ;
#7606=CARTESIAN_POINT ( 'NONE',  ( 26.27730496000000215, 9.202811183099997905, 229.9172022029999880 ) ) ;
#7607=CARTESIAN_POINT ( 'NONE',  ( -14.81011783459999975, -10.71728792430000077, 230.6999999999999886 ) ) ;
#7618=AXIS2_PLACEMENT_3D ( 'NONE', #5531, #22075, #982 ) ;
#7634=CARTESIAN_POINT ( 'NONE',  ( -11.95978252129999930, -1.610295041749999934, 231.9999989789999972 ) ) ;
#7674=EDGE_CURVE ( 'NONE', #18191, #5647, #8168, .T. ) ;
#7678=CARTESIAN_POINT ( 'NONE',  ( -26.78802611780000120, 9.366666170069999353, 229.2930777859999978 ) ) ;
#7711=CARTESIAN_POINT ( 'NONE',  ( -28.50000000000000000, 1.776356839399999922E-14, 222.0000000000000000 ) ) ;
#7716=AXIS2_PLACEMENT_3D ( 'NONE', #6186, #23355, #1795 ) ;
#7744=CARTESIAN_POINT ( 'NONE',  ( 2.131628207279999844E-14, 1.421085471519999843E-14, 230.7531949689999919 ) ) ;
#7751=CARTESIAN_POINT ( 'NONE',  ( 26.63983911210000244, 10.51862255760000053, 222.0000000000000000 ) ) ;
#7756=CARTESIAN_POINT ( 'NONE',  ( 24.33692359859999854, 13.51547608080000096, 229.9171999149999692 ) ) ;
#7771=AXIS2_PLACEMENT_3D ( 'NONE', #11283, #20886, #9064 ) ;
#7784=CARTESIAN_POINT ( 'NONE',  ( -5.114250173089999407, -17.43050732989999929, 231.6999999999999886 ) ) ;
#7785=ORIENTED_EDGE ( 'NONE', *, *, #4851, .F. ) ;
#7788=CARTESIAN_POINT ( 'NONE',  ( -11.39200449410000004, 4.622831274389999301, 232.6627643349999914 ) ) ;
#7791=CARTESIAN_POINT ( 'NONE',  ( -4.374602998565779721, 11.28407061768234954, 232.0000000000051443 ) ) ;
#7805=CARTESIAN_POINT ( 'NONE',  ( 24.10986967230000033, -13.84040926149999962, 226.0986570600000221 ) ) ;
#7818=CARTESIAN_POINT ( 'NONE',  ( 11.98808650430000000, -2.924528239270000274, 232.6627648150000027 ) ) ;
#7821=CARTESIAN_POINT ( 'NONE',  ( 26.80000000000000071, -6.039613253960000872E-14, 230.6999999999999886 ) ) ;
#7828=CARTESIAN_POINT ( 'NONE',  ( -24.07583586439999834, -13.90018868249999962, 226.1000014189999945 ) ) ;
#7832=CARTESIAN_POINT ( 'NONE',  ( -19.41565715145875615, 19.99999633038200741, 230.3176857765022874 ) ) ;
#7846=CARTESIAN_POINT ( 'NONE',  ( 23.74337837439999888, -14.46065164910000078, 225.9012998019999827 ) ) ;
#7858=FACE_OUTER_BOUND ( 'NONE', #27854, .T. ) ;
#7887=CARTESIAN_POINT ( 'NONE',  ( -20.30396346370000060, 20.00000000000000000, 227.0000000000000000 ) ) ;
#7888=B_SPLINE_CURVE_WITH_KNOTS ( 'NONE', 1,
 ( #23150, #18569 ),
 .UNSPECIFIED., .F., .F.,
 ( 2, 2 ),
 ( -4.314404719430000596E-12, 0.7012472868949999327 ),
 .UNSPECIFIED. ) ;
#7891=CARTESIAN_POINT ( 'NONE',  ( 23.51325844009999955, -14.83130343779999905, 224.7916311099999973 ) ) ;
#7897=CARTESIAN_POINT ( 'NONE',  ( -0.2873368412495915791, -28.49911791804343153, 223.9262120796962563 ) ) ;
#7925=CARTESIAN_POINT ( 'NONE',  ( -13.47758776899999944, -27.06128935389999768, 229.9172011129999760 ) ) ;
#7935=CARTESIAN_POINT ( 'NONE',  ( 18.31087175629999919, 19.88197256460000162, 229.9783849850000195 ) ) ;
#7971=CARTESIAN_POINT ( 'NONE',  ( -0.6521609807820000215, -27.79292263629999837, 224.0990923460000204 ) ) ;
#7984=CARTESIAN_POINT ( 'NONE',  ( -18.15901341782211276, 19.99997668335234735, 230.6866300220142421 ) ) ;
#7986=DIRECTION ( 'NONE',  ( 0.000000000000000000, 0.000000000000000000, -1.000000000000000000 ) ) ;
#8001=CARTESIAN_POINT ( 'NONE',  ( 24.62873585949999722, -14.34148440729999940, 226.0959678990000157 ) ) ;
#8008=CARTESIAN_POINT ( 'NONE',  ( -21.81244463630000396, 17.27887638289999828, 224.0000000000000000 ) ) ;
#8042=CARTESIAN_POINT ( 'NONE',  ( 26.05511440549999946, -14.93230011260000012, 222.0000000000000000 ) ) ;
#8044=AXIS2_PLACEMENT_3D ( 'NONE', #22963, #25647, #8466 ) ;
#8055=CARTESIAN_POINT ( 'NONE',  ( -22.19203486339999998, 17.78346196859999750, 230.2432540810000319 ) ) ;
#8058=CARTESIAN_POINT ( 'NONE',  ( 13.33996102200000244, -12.49969090709999975, 230.6999999999999886 ) ) ;
#8065=B_SPLINE_CURVE_WITH_KNOTS ( 'NONE', 5,
 ( #5511, #17765, #14966, #10244, #3302, #22515, #10397, #809, #19988 ),
 .UNSPECIFIED., .F., .F.,
 ( 6, 3, 6 ),
 ( 8.011061266649999624, 9.372199858680000162, 10.73333845069999981 ),
 .UNSPECIFIED. ) ;
#8092=CARTESIAN_POINT ( 'NONE',  ( -3.378474373710000034, -11.51459555979999827, 232.0000000000000000 ) ) ;
#8097=CARTESIAN_POINT ( 'NONE',  ( -23.50695179570000093, -14.84192241259999889, 225.0000014190000002 ) ) ;
#8099=CARTESIAN_POINT ( 'NONE',  ( 28.49999999959999641, 10.47094317839999889, 229.0000000000000000 ) ) ;
#8116=B_SPLINE_CURVE_WITH_KNOTS ( 'NONE', 3,
 ( #9415, #11937, #21545, #26571, #16808, #26422, #5011, #21860, #11631, #11787, #23606, #4864 ),
 .UNSPECIFIED., .F., .F.,
 ( 4, 2, 2, 2, 2, 4 ),
 ( 0.000000000000000000, 0.2499999999999725775, 0.4999999999999451550, 0.6249999999999481526, 0.7499999999999512612, 1.000000000000000000 ),
 .UNSPECIFIED. ) ;
#8126=EDGE_CURVE ( 'NONE', #30938, #10989, #13138, .T. ) ;
#8135=CARTESIAN_POINT ( 'NONE',  ( -27.71720220739999974, -1.978379369349999957E-11, 229.4485730569999760 ) ) ;
#8140=ORIENTED_EDGE ( 'NONE', *, *, #28038, .T. ) ;
#8167=FACE_OUTER_BOUND ( 'NONE', #26322, .T. ) ;
#8168=B_SPLINE_CURVE_WITH_KNOTS ( 'NONE', 1,
 ( #26483, #4927 ),
 .UNSPECIFIED., .F., .F.,
 ( 2, 2 ),
 ( -9.355471259890000464E-07, 0.7003637394550000783 ),
 .UNSPECIFIED. ) ;
#8186=CARTESIAN_POINT ( 'NONE',  ( 27.04041630560000087, 4.566211381850000528, 230.6999999999999886 ) ) ;
#8193=CARTESIAN_POINT ( 'NONE',  ( -0.3831792618880000556, -28.49793954440000121, 226.0423263479999889 ) ) ;
#8203=CARTESIAN_POINT ( 'NONE',  ( -18.17096239019999970, 20.37181511190000194, 230.6577119970000069 ) ) ;
#8205=CARTESIAN_POINT ( 'NONE',  ( -13.75032424529999986, -27.60893268180000248, 222.0000000000000000 ) ) ;
#8206=CARTESIAN_POINT ( 'NONE',  ( -19.80526803560000104, 19.50877411510000314, 227.0000000000000000 ) ) ;
#8226=CARTESIAN_POINT ( 'NONE',  ( -27.77512470389999777, -10.20462277120000039, 229.2930777930000090 ) ) ;
#8228=CARTESIAN_POINT ( 'NONE',  ( -27.03927855759999943, -7.087469713119999959, 222.0000000000000000 ) ) ;
#8238=FACE_OUTER_BOUND ( 'NONE', #29224, .T. ) ;
#8240=STYLED_ITEM ( 'NONE', ( #17546 ), #21535 ) ;
#8241=VECTOR ( 'NONE', #13416, 1000.000000000000114 ) ;
#8266=CARTESIAN_POINT ( 'NONE',  ( 18.26224557211887145, 20.00000411661503108, 230.6762370528171004 ) ) ;
#8277=CARTESIAN_POINT ( 'NONE',  ( -0.4702726640079999965, -27.79650200060000031, 223.9974845609999932 ) ) ;
#8283=CARTESIAN_POINT ( 'NONE',  ( -24.68204616399999907, -14.25020164319999871, 226.1000014189999945 ) ) ;
#8291=CARTESIAN_POINT ( 'NONE',  ( -19.33022990401857300, 20.00006911879202320, 230.3642850961209660 ) ) ;
#8294=ORIENTED_EDGE ( 'NONE', *, *, #18911, .F. ) ;
#8303=EDGE_LOOP ( 'NONE', ( #19560, #26626, #4810, #17387 ) ) ;
#8307=CARTESIAN_POINT ( 'NONE',  ( 2.131628207279999844E-14, 1.421085471519999843E-14, 231.6999999999999886 ) ) ;
#8321=CARTESIAN_POINT ( 'NONE',  ( 3.550686850769999806E-05, -28.50022181210000127, 226.1000014189999945 ) ) ;
#8328=DIRECTION ( 'NONE',  ( -0.2665630446479613780, -0.9085064176298685013, -0.3218077568259533061 ) ) ;
#8331=B_SPLINE_CURVE_WITH_KNOTS ( 'NONE', 5,
 ( #7027, #30791, #28117, #28427, #28729, #6861, #16463, #111, #26077, #25768, #16616, #26223, #2316, #23717, #12056 ),
 .UNSPECIFIED., .F., .F.,
 ( 6, 3, 3, 3, 6 ),
 ( 0.000000000000000000, 0.1000000000005726170, 0.4000000000022904678, 0.7000000000005726086, 1.000000000000000000 ),
 .UNSPECIFIED. ) ;
#8334=ORIENTED_EDGE ( 'NONE', *, *, #4064, .F. ) ;
#8340=CARTESIAN_POINT ( 'NONE',  ( 23.93626153989999850, 13.29299652659999964, 230.6999999999999886 ) ) ;
#8358=CARTESIAN_POINT ( 'NONE',  ( -23.94309786570000043, 13.28188914049999880, 230.6999999999999886 ) ) ;
#8362=CARTESIAN_POINT ( 'NONE',  ( 17.50139513559999926, -5.282204535990000061, 230.6999999999999886 ) ) ;
#8370=CARTESIAN_POINT ( 'NONE',  ( 21.02350438529999721, 19.26967166389999875, 225.9999999149999894 ) ) ;
#8382=CARTESIAN_POINT ( 'NONE',  ( -27.53132592969999948, -10.11505073740000071, 229.7313259299999686 ) ) ;
#8418=EDGE_LOOP ( 'NONE', ( #16782, #8893, #12386, #1078 ) ) ;
#8429=CARTESIAN_POINT ( 'NONE',  ( -0.8057362888000000334, -27.78873281839999976, 224.2403608809999866 ) ) ;
#8433=CARTESIAN_POINT ( 'NONE',  ( 1.092747331740645533, -27.77868070731554795, 225.1457540162050748 ) ) ;
#8444=CARTESIAN_POINT ( 'NONE',  ( -18.12672911204381165, 19.99995619754870901, 230.6891754141428237 ) ) ;
#8450=EDGE_LOOP ( 'NONE', ( #19044, #406, #15581, #13701 ) ) ;
#8452=CIRCLE ( 'NONE', #14184, 18.16530045500000057 ) ;
#8456=ORIENTED_EDGE ( 'NONE', *, *, #5021, .F. ) ;
#8466=DIRECTION ( 'NONE',  ( 0.2815395311429196301, 0.9595496299847262600, 0.000000000000000000 ) ) ;
#8471=CARTESIAN_POINT ( 'NONE',  ( 3.550686847520000117E-05, -28.50022181210000127, 223.9000014189999774 ) ) ;
#8481=CARTESIAN_POINT ( 'NONE',  ( 20.30405755279999980, 20.00000000000000000, 227.7999999360000061 ) ) ;
#8491=CARTESIAN_POINT ( 'NONE',  ( -25.22069443620000229, -13.27363204220000092, 224.7915656799999908 ) ) ;
#8499=ORIENTED_EDGE ( 'NONE', *, *, #50, .T. ) ;
#8501=ORIENTED_EDGE ( 'NONE', *, *, #50, .F. ) ;
#8503=CARTESIAN_POINT ( 'NONE',  ( 28.49999999979999998, -7.466149220249999274, 222.0000000000000000 ) ) ;
#8515=CARTESIAN_POINT ( 'NONE',  ( -27.44635497490000020, 9.596816764059999727, 229.4982322489999831 ) ) ;
#8519=CARTESIAN_POINT ( 'NONE',  ( -23.10935684530000245, -20.42749692129999772, 229.0000000000000000 ) ) ;
#8520=CARTESIAN_POINT ( 'NONE',  ( -4.340019564239999461, -26.72143554420000200, 230.6999999999999886 ) ) ;
#8544=CARTESIAN_POINT ( 'NONE',  ( -27.79999999999999716, 2.355804440410000085E-11, 229.1414213560000235 ) ) ;
#8554=CARTESIAN_POINT ( 'NONE',  ( 19.49298387170000169, 19.58648673140000440, 229.5592795560000070 ) ) ;
#8556=CARTESIAN_POINT ( 'NONE',  ( 24.10986967230000033, -13.84040926149999962, 223.9013457789999961 ) ) ;
#8577=CARTESIAN_POINT ( 'NONE',  ( 18.67857132407096188, 19.99999793005311943, 230.6030643836558340 ) ) ;
#8583=B_SPLINE_CURVE_WITH_KNOTS ( 'NONE', 1,
 ( #13431, #1803 ),
 .UNSPECIFIED., .F., .F.,
 ( 2, 2 ),
 ( -2.556331278550000249E-06, 0.7000000000009999335 ),
 .UNSPECIFIED. ) ;
#8609=ORIENTED_EDGE ( 'NONE', *, *, #19711, .F. ) ;
#8635=CARTESIAN_POINT ( 'NONE',  ( 0.6521647004709999473, -27.79285400239999859, 224.0990955869999937 ) ) ;
#8642=EDGE_CURVE ( 'NONE', #1273, #15181, #1872, .T. ) ;
#8645=LINE ( 'NONE', #13377, #15756 ) ;
#8659=B_SPLINE_CURVE_WITH_KNOTS ( 'NONE', 5,
 ( #7458, #9665, #30763, #86, #239, #19422 ),
 .UNSPECIFIED., .F., .F.,
 ( 6, 6 ),
 ( 0.000000000000000000, 21.63799706120000010 ),
 .UNSPECIFIED. ) ;
#8661=CARTESIAN_POINT ( 'NONE',  ( 5.114250173790000353, 17.43050733020000109, 230.6999999999999886 ) ) ;
#8668=CARTESIAN_POINT ( 'NONE',  ( -1.089818731930000117, -28.47945802909999813, 225.3102023309999993 ) ) ;
#8675=CARTESIAN_POINT ( 'NONE',  ( -24.62438106040000108, 13.65981548289999914, 230.5592437530000041 ) ) ;
#8680=CARTESIAN_POINT ( 'NONE',  ( 16.58809447609999665, 7.862979437299999041, 230.6999999999999886 ) ) ;
#8687=CARTESIAN_POINT ( 'NONE',  ( 21.71012070049999920, 18.50699920749999805, 224.9999999359999947 ) ) ;
#8695=EDGE_LOOP ( 'NONE', ( #3205, #13573, #20980, #24626, #17598 ) ) ;
#8701=CARTESIAN_POINT ( 'NONE',  ( 27.77512470400000311, -7.276253507709999901, 229.2930777930000090 ) ) ;
#8716=CARTESIAN_POINT ( 'NONE',  ( 24.30716200859999887, -13.49132717699999873, 223.9972514410000031 ) ) ;
#8727=CARTESIAN_POINT ( 'NONE',  ( 22.83442928010000017, 16.43389279790000046, 226.2000000000000171 ) ) ;
#8739=CARTESIAN_POINT ( 'NONE',  ( 18.94383107422812174, 20.00027397745331115, 230.5276813009044474 ) ) ;
#8749=ADVANCED_FACE ( 'NONE', ( #21060 ), #8907, .F. ) ;
#8755=VERTEX_POINT ( 'NONE', #17099 ) ;
#8760=CARTESIAN_POINT ( 'NONE',  ( -24.64674669160000064, -14.31123007319999907, 226.0986578890000089 ) ) ;
#8778=ORIENTED_EDGE ( 'NONE', *, *, #15831, .T. ) ;
#8795=B_SPLINE_CURVE_WITH_KNOTS ( 'NONE', 3,
 ( #24525, #29391, #10661, #10361, #29851, #22777, #29545, #17580, #3416, #5932, #5626, #7828 ),
 .UNSPECIFIED., .F., .F.,
 ( 4, 2, 2, 2, 2, 4 ),
 ( 0.000000000000000000, 0.1249999999999845124, 0.2499999999999690248, 0.4999999999999793499, 0.7499999999999896749, 1.000000000000000000 ),
 .UNSPECIFIED. ) ;
#8799=CARTESIAN_POINT ( 'NONE',  ( 1.099998580829999906, -27.77839262550000043, 225.0000014190000002 ) ) ;
#8810=CARTESIAN_POINT ( 'NONE',  ( -25.22658730140000216, -13.26242337740000110, 225.0000014190000002 ) ) ;
#8815=EDGE_CURVE ( 'NONE', #13541, #27946, #4461, .T. ) ;
#8820=CARTESIAN_POINT ( 'NONE',  ( -24.87138426050000106, -13.91768300640000078, 226.0425107039999943 ) ) ;
#8833=CARTESIAN_POINT ( 'NONE',  ( -27.79999999990000248, 3.326931647099999889, 222.0000000000000000 ) ) ;
#8841=CARTESIAN_POINT ( 'NONE',  ( 20.30405755279999980, 20.00000000000000000, 228.5999999789999890 ) ) ;
#8847=CARTESIAN_POINT ( 'NONE',  ( -24.73474822280000041, -14.15859640590000090, 226.0959706989999916 ) ) ;
#8853=ADVANCED_FACE ( 'NONE', ( #24189 ), #13951, .T. ) ;
#8861=CARTESIAN_POINT ( 'NONE',  ( 27.53132592980000126, -7.212385509899999825, 229.7313259299999686 ) ) ;
#8863=CARTESIAN_POINT ( 'NONE',  ( -14.53037274729999950, -23.87930420520000041, 222.0000000000000000 ) ) ;
#8875=PRODUCT_DEFINITION ( 'UNKNOWN', '', #17365, #3681 ) ;
#8884=CARTESIAN_POINT ( 'NONE',  ( 19.80538173169999894, 19.50875421069999760, 226.2000000000000171 ) ) ;
#8893=ORIENTED_EDGE ( 'NONE', *, *, #2892, .F. ) ;
#8907=B_SPLINE_SURFACE_WITH_KNOTS ( 'NONE', 5, 1, ( 
 ( #4529, #4214 ),
 ( #4063, #2173 ),
 ( #18681, #30660 ),
 ( #11764, #13817 ),
 ( #6875, #16328 ),
 ( #26092, #1703 ),
 ( #18531, #21368 ),
 ( #30964, #11304 ),
 ( #21207, #28282 ),
 ( #28133, #28602 ),
 ( #20905, #6571 ),
 ( #6723, #11610 ),
 ( #4370, #28443 ),
 ( #9394, #18997 ),
 ( #7042, #16632 ) ),
 .UNSPECIFIED., .F., .F., .F.,
 ( 6, 3, 3, 3, 6 ),
 ( 2, 2 ),
 ( 0.000000000000000000, 0.5239055192729999977, 1.047811038550000129, 1.571716557820000082, 1.746351730910000066 ),
 ( -0.7000000000009999335, 2.557302930970000000E-06 ),
 .UNSPECIFIED. ) ;
#8914=CARTESIAN_POINT ( 'NONE',  ( 19.76610007289999871, 19.51851078889999869, 229.2246588520000046 ) ) ;
#8949=CARTESIAN_POINT ( 'NONE',  ( 26.05511440539999768, -14.93230011240000010, 229.2404163060000144 ) ) ;
#8958=CARTESIAN_POINT ( 'NONE',  ( -1.419173379619999950E-06, -27.80022181310000207, 223.9000014189999774 ) ) ;
#8977=CARTESIAN_POINT ( 'NONE',  ( 18.94276922629999760, 21.23709851079999922, 229.4982322489999831 ) ) ;
#8978=ORIENTED_EDGE ( 'NONE', *, *, #30602, .F. ) ;
#8979=CARTESIAN_POINT ( 'NONE',  ( -24.46845037339999962, -13.19716075180000026, 225.7602695470000072 ) ) ;
#8987=CARTESIAN_POINT ( 'NONE',  ( -19.68707896189999929, 19.53815547089999782, 229.3695869349999725 ) ) ;
#8988=EDGE_CURVE ( 'NONE', #13739, #5647, #27742, .T. ) ;
#8996=CARTESIAN_POINT ( 'NONE',  ( -24.09883371379999772, -15.21565466309999870, 225.0000014190000002 ) ) ;
#8998=CARTESIAN_POINT ( 'NONE',  ( 25.22625794089999829, -13.26224522399999906, 225.0000014190000002 ) ) ;
#9021=CARTESIAN_POINT ( 'NONE',  ( 27.79999999980000069, -7.282770092329999834, 229.0000000000000000 ) ) ;
#9031=CARTESIAN_POINT ( 'NONE',  ( 24.68173674080000168, -14.25001227039999918, 223.9000014189999774 ) ) ;
#9035=CARTESIAN_POINT ( 'NONE',  ( -23.72449085899999943, 15.79286685369999788, 222.0000000000000000 ) ) ;
#9044=CARTESIAN_POINT ( 'NONE',  ( 19.80538173169999894, 19.50875421069999760, 229.0000000000000000 ) ) ;
#9051=SURFACE_STYLE_USAGE ( .BOTH. , #25748 ) ;
#9059=ORIENTED_EDGE ( 'NONE', *, *, #17231, .F. ) ;
#9064=DIRECTION ( 'NONE',  ( 1.000000000000000000, 0.000000000000000000, 0.000000000000000000 ) ) ;
#9071=CARTESIAN_POINT ( 'NONE',  ( 19.99469103059999853, 20.00000688379999758, 229.8491879540000014 ) ) ;
#9101=CARTESIAN_POINT ( 'NONE',  ( -23.69119896560000171, -20.94188573509999785, 229.0000000000000000 ) ) ;
#9103=CARTESIAN_POINT ( 'NONE',  ( 22.97596755210000197, 15.65128466780000061, 222.0000000000000000 ) ) ;
#9109=CARTESIAN_POINT ( 'NONE',  ( -24.12724309970000292, -13.81083407110000039, 223.9040321390000088 ) ) ;
#9119=CARTESIAN_POINT ( 'NONE',  ( -24.30742244220000003, -13.49161940279999961, 223.9971936000000028 ) ) ;
#9129=CARTESIAN_POINT ( 'NONE',  ( 5.689665389580000010, 17.26167590659999718, 230.6999999999999886 ) ) ;
#9136=CARTESIAN_POINT ( 'NONE',  ( -19.79257232079999795, 19.51192870039999860, 229.1494017060000203 ) ) ;
#9147=FACE_OUTER_BOUND ( 'NONE', #20506, .T. ) ;
#9153=CARTESIAN_POINT ( 'NONE',  ( -27.24857305720000156, 4.594528870269999565, 229.9172022069999741 ) ) ;
#9158=CARTESIAN_POINT ( 'NONE',  ( 25.17364887440000132, -13.36205984479999920, 225.5069763079999916 ) ) ;
#9159=CARTESIAN_POINT ( 'NONE',  ( 23.55447121679999967, 16.04539731370000055, 222.0000000000000000 ) ) ;
#9164=B_SPLINE_SURFACE_WITH_KNOTS ( 'NONE', 5, 1, ( 
 ( #21313, #25891 ),
 ( #30916, #9343 ),
 ( #18944, #1970 ),
 ( #9035, #13760 ),
 ( #11562, #26191 ),
 ( #6994, #20690 ),
 ( #13924, #18479 ),
 ( #16582, #18633 ),
 ( #4626, #21158 ),
 ( #23060, #6674 ),
 ( #6523, #28396 ),
 ( #11095, #30287 ) ),
 .UNSPECIFIED., .F., .F., .F.,
 ( 6, 3, 3, 6 ),
 ( 2, 2 ),
 ( 71.78637897720000183, 72.28968605440000772, 84.34526466259998756, 88.66823396320000938 ),
 ( -4.314404719430000596E-12, 0.7012472868949999327 ),
 .UNSPECIFIED. ) ;
#9170=CARTESIAN_POINT ( 'NONE',  ( 20.44762307379999910, -20.57851214589999955, 229.7313246180000021 ) ) ;
#9173=CARTESIAN_POINT ( 'NONE',  ( 28.50002393070000295, -0.8733865600460000156, 222.0000000000000000 ) ) ;
#9224=CARTESIAN_POINT ( 'NONE',  ( -0.8958568848300000331, -28.48628573779999940, 225.6801695290000112 ) ) ;
#9246=CARTESIAN_POINT ( 'NONE',  ( -24.09883371379999772, -15.21565466309999870, 225.0000014190000002 ) ) ;
#9249=CARTESIAN_POINT ( 'NONE',  ( -24.07583586439999834, -13.90018868249999962, 223.9000014189999774 ) ) ;
#9253=CARTESIAN_POINT ( 'NONE',  ( -27.56257419720000357, -10.12653142719999799, 230.5592437530000041 ) ) ;
#9257=CARTESIAN_POINT ( 'NONE',  ( -27.79999999999999716, -2.356913896269999927E-11, 224.8000000000000114 ) ) ;
#9262=CARTESIAN_POINT ( 'NONE',  ( -24.11017618899999704, -13.84060607850000046, 223.9013449680000178 ) ) ;
#9271=EDGE_LOOP ( 'NONE', ( #18914, #10534, #22295, #23003 ) ) ;
#9274=CARTESIAN_POINT ( 'NONE',  ( -24.11017618899999704, -13.84060607850000046, 223.9013449680000178 ) ) ;
#9290=CARTESIAN_POINT ( 'NONE',  ( -24.60124998910000116, -12.94761260449999973, 225.2084371580000095 ) ) ;
#9307=CARTESIAN_POINT ( 'NONE',  ( -23.83777999500000178, -14.30502388290000049, 226.0028091380000035 ) ) ;
#9313=CARTESIAN_POINT ( 'NONE',  ( -21.97984812610000205, 17.61343233899999916, 229.2930777540000236 ) ) ;
#9332=CARTESIAN_POINT ( 'NONE',  ( 24.58974021188865322, -12.96866346451374774, 225.2881025212954000 ) ) ;
#9333=CARTESIAN_POINT ( 'NONE',  ( -8.035257673360000297, -26.87837576509999593, 222.0000000000000000 ) ) ;
#9334=CARTESIAN_POINT ( 'NONE',  ( 1.127732790480000080, -28.47784299079999926, 225.1040528159999781 ) ) ;
#9339=CARTESIAN_POINT ( 'NONE',  ( -1.906343950897046113, -12.18129130007007888, 232.6627637558541437 ) ) ;
#9343=CARTESIAN_POINT ( 'NONE',  ( -23.03132590089999709, 15.56947127769999994, 222.0000000000000000 ) ) ;
#9386=CARTESIAN_POINT ( 'NONE',  ( 8.359832557563507294, -8.751033282714830719, 232.0000002394077683 ) ) ;
#9394=CARTESIAN_POINT ( 'NONE',  ( -24.66442003930000126, -14.28072947929999970, 223.9000014189999774 ) ) ;
#9407=CARTESIAN_POINT ( 'NONE',  ( 0.4162902733250000153, -12.33263093849999947, 232.6627648150000027 ) ) ;
#9411=CARTESIAN_POINT ( 'NONE',  ( 21.16705260759999874, -21.30254494150000255, 229.2404163060000144 ) ) ;
#9413=CARTESIAN_POINT ( 'NONE',  ( -24.62906106470000012, -14.34164290000000008, 223.9040321109999923 ) ) ;
#9415=CARTESIAN_POINT ( 'NONE',  ( -1.419173393149999842E-06, -27.80022181310000207, 226.1000014189999945 ) ) ;
#9453=CARTESIAN_POINT ( 'NONE',  ( -17.99591469510000152, 19.96082041680000074, 229.9999991770000065 ) ) ;
#9466=B_SPLINE_CURVE_WITH_KNOTS ( 'NONE', 1,
 ( #16727, #26190 ),
 .UNSPECIFIED., .F., .F.,
 ( 2, 2 ),
 ( -2.557302930970000000E-06, 0.7000000000009999335 ),
 .UNSPECIFIED. ) ;
#9467=CARTESIAN_POINT ( 'NONE',  ( 27.53132593009999951, 1.219166508230000085E-11, 229.7313259299999686 ) ) ;
#9468=CARTESIAN_POINT ( 'NONE',  ( 1.776356839399999922E-14, 0.000000000000000000, 232.6627637660000119 ) ) ;
#9477=CARTESIAN_POINT ( 'NONE',  ( 25.22036945370000183, -13.27344566769999901, 225.2083619149999834 ) ) ;
#9478=CARTESIAN_POINT ( 'NONE',  ( 22.97726876109999949, 16.89265187250000011, 222.9999999789999947 ) ) ;
#9482=EDGE_LOOP ( 'NONE', ( #25356, #19932, #27849, #29752 ) ) ;
#9484=ORIENTED_EDGE ( 'NONE', *, *, #8642, .T. ) ;
#9486=TOROIDAL_SURFACE ( 'NONE', #6469, 18.16530045470000232, 1.699999999999999956 ) ;
#9487=CARTESIAN_POINT ( 'NONE',  ( 28.50000000000000000, -5.921189464669998951E-16, 222.0000000000000000 ) ) ;
#9492=CARTESIAN_POINT ( 'NONE',  ( -12.74904032510000107, -25.66466679760000247, 222.0000000000000000 ) ) ;
#9493=CARTESIAN_POINT ( 'NONE',  ( 1.089891362629999971, -28.47934442809999922, 225.3101849020000031 ) ) ;
#9535=CARTESIAN_POINT ( 'NONE',  ( 24.43762869010000216, -14.66515636309999948, 223.9972528570000065 ) ) ;
#9543=CARTESIAN_POINT ( 'NONE',  ( -12.28060600210000075, -0.5788309733769999577, 232.6627643349999914 ) ) ;
#9546=CARTESIAN_POINT ( 'NONE',  ( -5.023648568049999596, -17.12171681569999748, 230.7531949689999919 ) ) ;
#9558=CARTESIAN_POINT ( 'NONE',  ( 24.60666743799999878, -12.93650359530000138, 225.1041818340000020 ) ) ;
#9567=CARTESIAN_POINT ( 'NONE',  ( 23.40936070919999779, 16.84772962260000284, 229.0000000000000000 ) ) ;
#9572=CARTESIAN_POINT ( 'NONE',  ( 8.417769050959998722, 8.647000318390000828, 231.9999991140000191 ) ) ;
#9576=CARTESIAN_POINT ( 'NONE',  ( 25.19810601000000361, -14.44114490489999980, 230.5592437530000041 ) ) ;
#9612=CARTESIAN_POINT ( 'NONE',  ( -19.29867024690000221, 19.63492390480000083, 229.6953880050000123 ) ) ;
#9634=EDGE_LOOP ( 'NONE', ( #13942, #14217, #27386, #19190 ) ) ;
#9648=ORIENTED_EDGE ( 'NONE', *, *, #14035, .T. ) ;
#9656=CARTESIAN_POINT ( 'NONE',  ( 27.54633501930000250, 4.750421692669999807, 222.0000000000000000 ) ) ;
#9661=CARTESIAN_POINT ( 'NONE',  ( 27.79999999999999716, -2.352589991099999975E-11, 229.1414213560000235 ) ) ;
#9662=CARTESIAN_POINT ( 'NONE',  ( -16.58808965729999940, -7.862989603470000866, 230.6999999999999886 ) ) ;
#9663=ORIENTED_EDGE ( 'NONE', *, *, #13520, .T. ) ;
#9665=CARTESIAN_POINT ( 'NONE',  ( 27.79999999980000069, 4.333901714429999608, 229.0000000000000000 ) ) ;
#9670=CARTESIAN_POINT ( 'NONE',  ( 19.31629274950000408, 18.68265037930000005, 230.6999999999999886 ) ) ;
#9688=DIRECTION ( 'NONE',  ( 0.9595496299847263710, -0.2815395311429191305, 0.000000000000000000 ) ) ;
#9692=CARTESIAN_POINT ( 'NONE',  ( -12.24209934469999972, 1.548575594009999890, 232.6627643349999914 ) ) ;
#9696=CARTESIAN_POINT ( 'NONE',  ( 24.49848005072939827, -13.14029679208924151, 224.3227009702077908 ) ) ;
#9715=EDGE_CURVE ( 'NONE', #5647, #15181, #22536, .T. ) ;
#9721=CARTESIAN_POINT ( 'NONE',  ( 3.441895620960000013, 11.73074934140000103, 232.6627648150000027 ) ) ;
#9731=CARTESIAN_POINT ( 'NONE',  ( -24.60699806910000120, -12.93667933180000063, 225.0000014190000002 ) ) ;
#9766=CARTESIAN_POINT ( 'NONE',  ( -23.62948527985757963, -14.64611956755585709, 224.3223991483396560 ) ) ;
#9782=ADVANCED_FACE ( 'NONE', ( #529 ), #28260, .F. ) ;
#9791=B_SPLINE_SURFACE_WITH_KNOTS ( 'NONE', 5, 1, ( 
 ( #24448, #2883 ),
 ( #28844, #29306 ),
 ( #26959, #9656 ),
 ( #5545, #14696 ),
 ( #7751, #7302 ),
 ( #16890, #12020 ),
 ( #29005, #29155 ),
 ( #17047, #24139 ),
 ( #4937, #10283 ) ),
 .UNSPECIFIED., .F., .F., .F.,
 ( 6, 3, 6 ),
 ( 2, 2 ),
 ( 0.000000000000000000, 12.04143823630000121, 16.88247121709999732 ),
 ( -3.785313009420000493E-15, 0.7017044499210000064 ),
 .UNSPECIFIED. ) ;
#9792=CARTESIAN_POINT ( 'NONE',  ( 24.73445225629999911, -14.15837998019999944, 226.0959682270000144 ) ) ;
#9800=CARTESIAN_POINT ( 'NONE',  ( -21.16705332919999805, 21.30254446269999846, 229.0000000000000000 ) ) ;
#9803=ORIENTED_EDGE ( 'NONE', *, *, #29891, .F. ) ;
#9810=ORIENTED_EDGE ( 'NONE', *, *, #22721, .F. ) ;
#9844=EDGE_CURVE ( 'NONE', #26590, #30960, #13980, .T. ) ;
#9851=CARTESIAN_POINT ( 'NONE',  ( -27.79999999999999716, -2.360757793890000105E-11, 229.0000000000000000 ) ) ;
#9852=CARTESIAN_POINT ( 'NONE',  ( 23.88690489929999927, -14.22221811490000043, 223.9575292099999899 ) ) ;
#9855=ADVANCED_FACE ( 'NONE', ( #10883 ), #4145, .T. ) ;
#9867=CARTESIAN_POINT ( 'NONE',  ( -24.69967241520000201, -14.21967358789999913, 223.9000014189999774 ) ) ;
#9869=CARTESIAN_POINT ( 'NONE',  ( 24.26025373720000289, -13.57556515269999942, 226.0424756639999941 ) ) ;
#9877=CARTESIAN_POINT ( 'NONE',  ( 22.97596755210000197, 15.65128466780000061, 222.0000000000000000 ) ) ;
#9881=CARTESIAN_POINT ( 'NONE',  ( 7.637033006139999358, 9.343723945229999828, 231.9999991140000191 ) ) ;
#9900=CARTESIAN_POINT ( 'NONE',  ( -18.50496050079999932, 20.74627092889999957, 229.1414212730000202 ) ) ;
#9969=CARTESIAN_POINT ( 'NONE',  ( -27.79999999999999716, -2.360778239559999931E-11, 229.0000000000000000 ) ) ;
#9977=CARTESIAN_POINT ( 'NONE',  ( 24.06257814289999786, 13.36313762839999875, 230.0000000000000000 ) ) ;
#10017=SURFACE_SIDE_STYLE ('',( #12519 ) ) ;
#10018=CARTESIAN_POINT ( 'NONE',  ( 28.50000000000000000, -5.921189464669998951E-16, 222.0000000000000000 ) ) ;
#10020=EDGE_CURVE ( 'NONE', #2003, #14789, #12686, .T. ) ;
#10040=CARTESIAN_POINT ( 'NONE',  ( 7.334768408830000475, -9.866585358490000957, 232.6627648150000027 ) ) ;
#10043=CARTESIAN_POINT ( 'NONE',  ( 28.04325408089999883, -7.346495424229999571, 230.2432540810000319 ) ) ;
#10059=CARTESIAN_POINT ( 'NONE',  ( -26.28018753080000280, 9.189075756099999381, 229.9172022029999880 ) ) ;
#10061=VERTEX_POINT ( 'NONE', #1993 ) ;
#10072=CARTESIAN_POINT ( 'NONE',  ( 20.05931974663578288, 19.99997412885312542, 229.7488604916501913 ) ) ;
#10108=ORIENTED_EDGE ( 'NONE', *, *, #16660, .F. ) ;
#10111=CARTESIAN_POINT ( 'NONE',  ( 27.04041630560000087, 3.053900541549999745E-14, 230.6999999999999886 ) ) ;
#10132=CARTESIAN_POINT ( 'NONE',  ( 21.31445244760000080, 17.08994352740000267, 230.0000000000000000 ) ) ;
#10142=B_SPLINE_SURFACE_WITH_KNOTS ( 'NONE', 5, 1, ( 
 ( #14185, #28339 ),
 ( #25991, #26295 ),
 ( #26146, #9136 ),
 ( #23788, #28795 ),
 ( #16686, #8987 ),
 ( #31016, #7097 ),
 ( #30559, #4740 ),
 ( #18740, #9612 ),
 ( #16383, #21584 ),
 ( #21427, #2073 ),
 ( #6787, #16226 ),
 ( #11512, #25840 ),
 ( #14034, #6626 ),
 ( #28497, #9453 ),
 ( #18587, #11664 ) ),
 .UNSPECIFIED., .F., .F., .F.,
 ( 6, 3, 3, 3, 6 ),
 ( 2, 2 ),
 ( 0.000000000000000000, 0.5777958940569999369, 1.155591788109999962, 2.022285629200000212, 2.888979470280000239 ),
 ( -1.118726812310000082E-05, 0.7031447686210000603 ),
 .UNSPECIFIED. ) ;
#10179=CARTESIAN_POINT ( 'NONE',  ( 24.73445225629999911, -14.15837998019999944, 226.0959682270000144 ) ) ;
#10192=B_SPLINE_CURVE_WITH_KNOTS ( 'NONE', 5,
 ( #12388, #138, #2492, #7050, #9567, #16640 ),
 .UNSPECIFIED., .F., .F.,
 ( 6, 6 ),
 ( 0.000000000000000000, 21.97608269730000075 ),
 .UNSPECIFIED. ) ;
#10193=CARTESIAN_POINT ( 'NONE',  ( 4.917756447549999521, 10.96637803540000000, 231.9999991140000191 ) ) ;
#10209=CARTESIAN_POINT ( 'NONE',  ( -18.94791452757604944, 20.00033874320078908, 230.5288124007003887 ) ) ;
#10220=EDGE_CURVE ( 'NONE', #30960, #24425, #18440, .T. ) ;
#10229=CARTESIAN_POINT ( 'NONE',  ( 24.68173674080000168, -14.25001227039999918, 226.1000014189999945 ) ) ;
#10240=CARTESIAN_POINT ( 'NONE',  ( 1.099998490678698593, -27.77839035186433136, 225.0734570122248215 ) ) ;
#10244=CARTESIAN_POINT ( 'NONE',  ( -27.56257419730000180, -2.940926349879999851E-14, 230.5592437530000041 ) ) ;
#10266=CARTESIAN_POINT ( 'NONE',  ( 28.50000000000000000, 3.195004098709999527E-14, 229.2404163060000144 ) ) ;
#10279=CARTESIAN_POINT ( 'NONE',  ( -0.8892886897209191233, -28.48641921395686794, 224.3203319190939737 ) ) ;
#10281=STYLED_ITEM ( 'NONE', ( #23396 ), #2064 ) ;
#10283=CARTESIAN_POINT ( 'NONE',  ( 22.97596219000000062, 15.65128142029999836, 222.0000000000000000 ) ) ;
#10287=CARTESIAN_POINT ( 'NONE',  ( 25.98110156819999972, 9.099016333859999861, 230.0000000000000000 ) ) ;
#10308=CARTESIAN_POINT ( 'NONE',  ( -22.52168649520000088, -19.90806591850000018, 229.9751242030000071 ) ) ;
#10315=DIRECTION ( 'NONE',  ( 0.9002473904559572526, -0.4353787270609801308, 0.000000000000000000 ) ) ;
#10317=CARTESIAN_POINT ( 'NONE',  ( 19.80538212960000166, 19.50875458629999670, 229.0000000010000178 ) ) ;
#10324=CARTESIAN_POINT ( 'NONE',  ( -11.76276068685807985, -2.846903954059027519, 232.0000000000047748 ) ) ;
#10346=CARTESIAN_POINT ( 'NONE',  ( -14.09657507470000226, -28.30410041510000241, 229.0000000000000000 ) ) ;
#10361=CARTESIAN_POINT ( 'NONE',  ( -23.52636877871646348, -14.81113159432834081, 225.2882641545094486 ) ) ;
#10393=CARTESIAN_POINT ( 'NONE',  ( 0.5493986535500280377, -27.79508000654526967, 225.9641420709400279 ) ) ;
#10397=CARTESIAN_POINT ( 'NONE',  ( -28.45771199730000234, -1.783000543380000178E-14, 229.4982322489999831 ) ) ;
#10401=CARTESIAN_POINT ( 'NONE',  ( 1.127732790480000080, -28.47784299079999926, 225.0000014190000002 ) ) ;
#10415=ADVANCED_FACE ( 'NONE', ( #3210 ), #30531, .T. ) ;
#10427=CARTESIAN_POINT ( 'NONE',  ( 23.50666810109999716, -14.84174128299999929, 225.0000014190000002 ) ) ;
#10435=CARTESIAN_POINT ( 'NONE',  ( -25.05382009470000071, 13.89803701039999950, 230.2432540810000319 ) ) ;
#10439=CARTESIAN_POINT ( 'NONE',  ( 27.53132592989999949, 4.649109393739999874, 229.7313259299999686 ) ) ;
#10448=VERTEX_POINT ( 'NONE', #30593 ) ;
#10462=CARTESIAN_POINT ( 'NONE',  ( -28.50002393070000295, -2.434994504239999635, 222.0000000000000000 ) ) ;
#10483=( LENGTH_UNIT ( ) NAMED_UNIT ( * ) SI_UNIT ( .MILLI., .METRE. ) );
#10505=CARTESIAN_POINT ( 'NONE',  ( -1.087696845100000198, -27.77899371300000197, 224.7918862260000026 ) ) ;
#10519=CARTESIAN_POINT ( 'NONE',  ( -18.02784043102035483, 19.99990957752277509, 230.6954974467259376 ) ) ;
#10534=ORIENTED_EDGE ( 'NONE', *, *, #10220, .F. ) ;
#10575=CARTESIAN_POINT ( 'NONE',  ( -20.30396346370000060, 20.00000000000000000, 227.3999999999999773 ) ) ;
#10578=CARTESIAN_POINT ( 'NONE',  ( 23.50666810109999716, -14.84174128299999929, 224.8958160969999938 ) ) ;
#10586=CARTESIAN_POINT ( 'NONE',  ( -28.35924375240000117, 4.781805056509999652, 229.7625741969999922 ) ) ;
#10589=FACE_BOUND ( 'NONE', #27978, .T. ) ;
#10590=CARTESIAN_POINT ( 'NONE',  ( -9.014669513459999450, -25.43090265169999853, 230.6999999999999886 ) ) ;
#10610=CARTESIAN_POINT ( 'NONE',  ( -27.54633509470000163, -4.750421057000000502, 222.0000000000000000 ) ) ;
#10621=CARTESIAN_POINT ( 'NONE',  ( -23.69119896570000350, -20.94188573499999961, 222.0000000000000000 ) ) ;
#10633=ADVANCED_FACE ( 'NONE', ( #24899 ), #354, .F. ) ;
#10642=CARTESIAN_POINT ( 'NONE',  ( 19.88997495436197482, 20.00029480896879974, 229.9620880754783911 ) ) ;
#10652=CARTESIAN_POINT ( 'NONE',  ( -0.03443693864410000277, -27.80022362959999782, 223.9000014189999774 ) ) ;
#10661=CARTESIAN_POINT ( 'NONE',  ( -23.51084008381386070, -14.83576737699261727, 225.1458431688038218 ) ) ;
#10665=CARTESIAN_POINT ( 'NONE',  ( -18.59970865813222218, 20.00000695728539668, 230.6210579144432984 ) ) ;
#10666=CARTESIAN_POINT ( 'NONE',  ( -27.79999999980000069, 4.687507935210000198, 229.1414213560000235 ) ) ;
#10679=ORIENTED_EDGE ( 'NONE', *, *, #20847, .T. ) ;
#10716=CARTESIAN_POINT ( 'NONE',  ( 27.04365979920000029, 9.471113331109998867, 230.2432540810000319 ) ) ;
#10719=CARTESIAN_POINT ( 'NONE',  ( -23.69119896570000350, -20.94188573499999961, 222.0000000000000000 ) ) ;
#10733=CARTESIAN_POINT ( 'NONE',  ( -28.45771199730000234, -1.047388408700000119E-14, 229.4982322489999831 ) ) ;
#10737=CARTESIAN_POINT ( 'NONE',  ( -0.1718244463979999859, -18.28023999129999666, 230.6999999999999886 ) ) ;
#10776=CARTESIAN_POINT ( 'NONE',  ( 3.441895497200000431, 11.73074891959999988, 232.6627635220000059 ) ) ;
#10787=CARTESIAN_POINT ( 'NONE',  ( 27.79999999990000248, 4.333901782529999025, 223.3999999999999773 ) ) ;
#10800=AXIS2_PLACEMENT_3D ( 'NONE', #24838, #7986, #3270 ) ;
#10802=CARTESIAN_POINT ( 'NONE',  ( 18.71271765012262378, 20.00001436454239112, 230.5947203350884820 ) ) ;
#10808=CARTESIAN_POINT ( 'NONE',  ( -28.50000000000000000, -5.684341886079999373E-14, 229.0000000000000000 ) ) ;
#10816=CARTESIAN_POINT ( 'NONE',  ( -0.8738876050350000702, -27.78662806160000187, 224.3198333100000070 ) ) ;
#10823=B_SPLINE_CURVE_WITH_KNOTS ( 'NONE', 1,
 ( #28974, #22059 ),
 .UNSPECIFIED., .F., .F.,
 ( 2, 2 ),
 ( -2.556023926959999973E-06, 0.7000000000009999335 ),
 .UNSPECIFIED. ) ;
#10870=CARTESIAN_POINT ( 'NONE',  ( 0.4821455017210000138, -28.49635764770000179, 223.9974824469999817 ) ) ;
#10883=FACE_OUTER_BOUND ( 'NONE', #18999, .T. ) ;
#10886=CARTESIAN_POINT ( 'NONE',  ( -20.30396346370000060, 20.00000000000000000, 229.0000000000000000 ) ) ;
#10897=CARTESIAN_POINT ( 'NONE',  ( -25.33612502140000089, 14.05463924120000030, 229.7625741969999922 ) ) ;
#10900=CARTESIAN_POINT ( 'NONE',  ( 25.41516571979999739, -14.56554164990000011, 229.0000000000000000 ) ) ;
#10901=CARTESIAN_POINT ( 'NONE',  ( 26.30683953509999640, -5.612727362360000249, 230.6999999999999886 ) ) ;
#10910=CARTESIAN_POINT ( 'NONE',  ( 2.131628207279999844E-14, 1.421085471519999843E-14, 231.6999999999999886 ) ) ;
#10933=CARTESIAN_POINT ( 'NONE',  ( 24.60092358069999818, -12.94742893959999819, 224.7916409239999780 ) ) ;
#10935=CARTESIAN_POINT ( 'NONE',  ( -28.49999999970000175, -10.47094308429999998, 222.0000000000000000 ) ) ;
#10943=CARTESIAN_POINT ( 'NONE',  ( 26.95545381250000361, 8.667969360499998999, 229.0000000000000000 ) ) ;
#10961=CARTESIAN_POINT ( 'NONE',  ( 23.88690489929999927, -14.22221811490000043, 226.0424736289999714 ) ) ;
#10973=CARTESIAN_POINT ( 'NONE',  ( 1.041496722224801719, -27.78066294026401906, 225.3591738694975675 ) ) ;
#10989=VERTEX_POINT ( 'NONE', #11317 ) ;
#10995=VERTEX_POINT ( 'NONE', #30516 ) ;
#11015=CARTESIAN_POINT ( 'NONE',  ( 0.8959394325020000327, -28.48619164239999790, 224.3198498209999912 ) ) ;
#11029=CARTESIAN_POINT ( 'NONE',  ( -25.22658730140000216, -13.26242337740000110, 224.8957833819999621 ) ) ;
#11042=CARTESIAN_POINT ( 'NONE',  ( -24.55564696219999732, -13.03410599059999875, 225.5071265450000055 ) ) ;
#11048=CARTESIAN_POINT ( 'NONE',  ( -0.8259893078309999970, -28.48844349870000059, 225.7596419580000315 ) ) ;
#11055=CARTESIAN_POINT ( 'NONE',  ( -28.50000000000000000, -3.445280580419999703E-14, 229.2404163060000144 ) ) ;
#11057=CARTESIAN_POINT ( 'NONE',  ( -23.95524095760000094, -14.10746636989999914, 226.0798679369999888 ) ) ;
#11058=CARTESIAN_POINT ( 'NONE',  ( 25.41516571979999739, -14.56554165020000013, 222.0000000000000000 ) ) ;
#11059=CARTESIAN_POINT ( 'NONE',  ( 0.5020148408599999224, -26.94192660829999753, 230.6999999999999886 ) ) ;
#11072=ORIENTED_EDGE ( 'NONE', *, *, #16426, .T. ) ;
#11081=CARTESIAN_POINT ( 'NONE',  ( 27.09307779329999732, -7.097577590990000296, 229.9751247039999953 ) ) ;
#11084=FACE_OUTER_BOUND ( 'NONE', #30265, .T. ) ;
#11095=CARTESIAN_POINT ( 'NONE',  ( -28.50000000000000000, 9.769962616700000205E-15, 222.0000000000000000 ) ) ;
#11104=CARTESIAN_POINT ( 'NONE',  ( 19.80538173169999894, 19.50875421069999760, 223.3999999999999773 ) ) ;
#11114=CARTESIAN_POINT ( 'NONE',  ( 19.67543717097858291, 20.00025387898711671, 230.1474802616772308 ) ) ;
#11116=CARTESIAN_POINT ( 'NONE',  ( -17.83931601609999973, 20.00000000000000000, 230.0000000010000178 ) ) ;
#11118=CARTESIAN_POINT ( 'NONE',  ( 24.02382125689999981, -13.98923529139999999, 226.0959678990000157 ) ) ;
#11125=CARTESIAN_POINT ( 'NONE',  ( -0.3738033647229999645, -27.79799560440000050, 223.9576764909999724 ) ) ;
#11128=CARTESIAN_POINT ( 'NONE',  ( 28.50000000000000000, -2.380388045690000432E-15, 229.2404163060000144 ) ) ;
#11164=EDGE_CURVE ( 'NONE', #28749, #6979, #16755, .T. ) ;
#11165=CONICAL_SURFACE ( 'NONE', #4630, 11.99999999999999467, 1.243158134259999770 ) ;
#11168=CARTESIAN_POINT ( 'NONE',  ( 1.015231355539999880, -28.48218680760000154, 224.4935313260000100 ) ) ;
#11170=CARTESIAN_POINT ( 'NONE',  ( -23.55406855550000245, 16.04544956020000157, 222.0000000000000000 ) ) ;
#11178=CARTESIAN_POINT ( 'NONE',  ( -24.60124998910000116, -12.94761260449999973, 224.7915656799999908 ) ) ;
#11190=CARTESIAN_POINT ( 'NONE',  ( -24.58975347950000057, -12.96948186770000078, 225.3106485179999936 ) ) ;
#11202=CARTESIAN_POINT ( 'NONE',  ( 25.22625794089999829, -13.26224522399999906, 224.8958210039999983 ) ) ;
#11205=CARTESIAN_POINT ( 'NONE',  ( -23.88727024790000186, -14.22229899360000083, 226.0425106499999970 ) ) ;
#11209=CARTESIAN_POINT ( 'NONE',  ( 7.576768089039999765, -25.98941641389999901, 230.6999999999999886 ) ) ;
#11217=CARTESIAN_POINT ( 'NONE',  ( 26.96724923820000086, 10.13406330579999803, 222.0000000000000000 ) ) ;
#11220=CARTESIAN_POINT ( 'NONE',  ( -25.00949650969999993, -13.66806287920000074, 225.9014032059999977 ) ) ;
#11231=CARTESIAN_POINT ( 'NONE',  ( -13.75032424559999988, -27.60893268290000080, 229.1414204800000221 ) ) ;
#11234=CARTESIAN_POINT ( 'NONE',  ( -0.9536751402149999945, -27.93707515359999860, 222.0000000000000000 ) ) ;
#11235=B_SPLINE_CURVE_WITH_KNOTS ( 'NONE', 5,
 ( #11757, #13810, #6414, #11606, #21203, #13969 ),
 .UNSPECIFIED., .F., .F.,
 ( 6, 6 ),
 ( -2.000000000000000000, 0.000000000000000000 ),
 .UNSPECIFIED. ) ;
#11258=CARTESIAN_POINT ( 'NONE',  ( -28.49999999979999998, 7.466149641079999455, 222.0000000000000000 ) ) ;
#11283=CARTESIAN_POINT ( 'NONE',  ( 0.000000000000000000, 0.000000000000000000, 230.6999999999999886 ) ) ;
#11289=CARTESIAN_POINT ( 'NONE',  ( 19.80537707599999919, 19.50874960799999869, 229.0000000010000178 ) ) ;
#11291=CARTESIAN_POINT ( 'NONE',  ( -24.55841378230000061, -14.46270012129999927, 226.0798679369999888 ) ) ;
#11304=CARTESIAN_POINT ( 'NONE',  ( -23.74375282219999761, -14.46070769699999836, 224.0986003170000060 ) ) ;
#11317=CARTESIAN_POINT ( 'NONE',  ( 3.550686850769999806E-05, -28.50022181210000127, 226.1000014189999945 ) ) ;
#11322=CARTESIAN_POINT ( 'NONE',  ( 26.01645409420000021, -14.91014372119999898, 229.4982322489999831 ) ) ;
#11329=CARTESIAN_POINT ( 'NONE',  ( 0.4821455017210000138, -28.49635764770000179, 223.9974824469999817 ) ) ;
#11331=CARTESIAN_POINT ( 'NONE',  ( -25.47204932480000039, 13.22994448760000097, 222.0000000000000000 ) ) ;
#11342=ORIENTED_EDGE ( 'NONE', *, *, #19160, .F. ) ;
#11349=CARTESIAN_POINT ( 'NONE',  ( -24.68204616399999907, -14.25020164319999871, 226.1000014189999945 ) ) ;
#11366=CARTESIAN_POINT ( 'NONE',  ( -24.10559463919999956, -15.20494734660000091, 225.2084356629999888 ) ) ;
#11394=CARTESIAN_POINT ( 'NONE',  ( -25.53422772419999731, -11.61914357240000051, 222.0000000000000000 ) ) ;
#11401=CARTESIAN_POINT ( 'NONE',  ( 10.52451969703728096, -6.422810664934133662, 232.6627636643594599 ) ) ;
#11409=CARTESIAN_POINT ( 'NONE',  ( 26.80000000000000071, 4.525613202499999765, 230.0000000000000000 ) ) ;
#11419=SHAPE_REPRESENTATION_RELATIONSHIP ( 'NONE' , 'NONE' ,  #22833, #2064 ) ;
#11425=ORIENTED_EDGE ( 'NONE', *, *, #25216, .T. ) ;
#11443=CARTESIAN_POINT ( 'NONE',  ( 19.80537707610000098, 19.50874960790000046, 229.0739602739999725 ) ) ;
#11449=AXIS2_PLACEMENT_3D ( 'NONE', #7744, #18819, #15145 ) ;
#11454=CARTESIAN_POINT ( 'NONE',  ( 5.114250173089999407, 17.43050732989999929, 231.6999999999999886 ) ) ;
#11472=CARTESIAN_POINT ( 'NONE',  ( -5.359734053730000447, -10.98902024870000105, 232.6627648150000027 ) ) ;
#11476=CARTESIAN_POINT ( 'NONE',  ( 5.135309658569999769, -30.28532181790000166, 230.6577119970000069 ) ) ;
#11483=CARTESIAN_POINT ( 'NONE',  ( 3.550686846709999450E-05, -28.50022181210000127, 223.9000014189999774 ) ) ;
#11503=CARTESIAN_POINT ( 'NONE',  ( 7.368918569919999939, 16.61433718970000228, 230.6999999999999886 ) ) ;
#11512=CARTESIAN_POINT ( 'NONE',  ( -18.41918783629999723, 20.00000925869999691, 230.6632488119999778 ) ) ;
#11528=CARTESIAN_POINT ( 'NONE',  ( -25.84755624059999946, 9.037785233839999322, 230.0000000000000000 ) ) ;
#11559=ORIENTED_EDGE ( 'NONE', *, *, #26804, .T. ) ;
#11562=CARTESIAN_POINT ( 'NONE',  ( -25.12323886820000141, 13.67941525610000042, 222.0000000000000000 ) ) ;
#11563=CARTESIAN_POINT ( 'NONE',  ( 0.8057459563030000549, -27.78864806999999715, 225.7596297540000023 ) ) ;
#11573=ADVANCED_FACE ( 'NONE', ( #24859 ), #4939, .T. ) ;
#11583=CARTESIAN_POINT ( 'NONE',  ( -19.49313842129999941, 19.58644462790000063, 229.5590894759999969 ) ) ;
#11596=FACE_OUTER_BOUND ( 'NONE', #4825, .T. ) ;
#11598=CARTESIAN_POINT ( 'NONE',  ( 0.2766207017872922003, 12.09920997781417107, 232.0000000000052864 ) ) ;
#11606=CARTESIAN_POINT ( 'NONE',  ( -20.30396346370000060, 20.00000000000000000, 228.1999999999999886 ) ) ;
#11607=DIRECTION ( 'NONE',  ( 0.2815395311429191305, 0.9595496299847262600, 0.000000000000000000 ) ) ;
#11610=CARTESIAN_POINT ( 'NONE',  ( -24.02415253779999915, -13.98938335050000070, 223.9040321109999923 ) ) ;
#11622=CARTESIAN_POINT ( 'NONE',  ( -3.862368227480000193, -11.41372166100000207, 231.9999991140000191 ) ) ;
#11626=CARTESIAN_POINT ( 'NONE',  ( -27.56257419730000180, 3.552713678799999608E-15, 230.5592437530000041 ) ) ;
#11627=B_SPLINE_CURVE_WITH_KNOTS ( 'NONE', 3,
 ( #2931, #4983, #24032, #2476, #12066, #14742, #9386, #21825, #19306, #24338, #7036, #14594, #21362, #28900, #7497, #2782, #26234, #11908 ),
 .UNSPECIFIED., .F., .F.,
 ( 4, 2, 2, 2, 2, 2, 2, 2, 4 ),
 ( 0.000000000000000000, 0.1250000000000000555, 0.2500000000000001110, 0.3750000000000001665, 0.5000000000000001110, 0.6250000000000001110, 0.7500000000000001110, 0.8750000000000000000, 1.000000000000000000 ),
 .UNSPECIFIED. ) ;
#11631=CARTESIAN_POINT ( 'NONE',  ( -0.9837773765372604950, -27.78287111172183899, 225.4958527047016617 ) ) ;
#11635=CARTESIAN_POINT ( 'NONE',  ( -24.39524108170000360, -13.33235248870000156, 224.0985996330000205 ) ) ;
#11657=CARTESIAN_POINT ( 'NONE',  ( -24.69967241520000201, -14.21967358789999913, 226.1000014189999945 ) ) ;
#11664=CARTESIAN_POINT ( 'NONE',  ( -17.83931601680000156, 20.00000000000000000, 229.9999991770000065 ) ) ;
#11674=CARTESIAN_POINT ( 'NONE',  ( -23.74375282219999761, -14.46070769699999836, 225.9014025209999943 ) ) ;
#11678=VERTEX_POINT ( 'NONE', #17903 ) ;
#11680=CARTESIAN_POINT ( 'NONE',  ( -21.78691859319999935, 17.45882806430000045, 229.7313258739999924 ) ) ;
#11685=CARTESIAN_POINT ( 'NONE',  ( 25.22625794089999829, -13.26224522399999906, 225.0000014190000002 ) ) ;
#11688=VERTEX_POINT ( 'NONE', #22959 ) ;
#11698=CARTESIAN_POINT ( 'NONE',  ( 24.63023943419999995, -14.11569779149999881, 230.0000000000000000 ) ) ;
#11700=CARTESIAN_POINT ( 'NONE',  ( 24.05322775159999793, -15.76571806769999995, 222.0000000000000000 ) ) ;
#11707=CARTESIAN_POINT ( 'NONE',  ( 2.900346228477644228, -11.98357204604639392, 232.6627637253559442 ) ) ;
#11727=CARTESIAN_POINT ( 'NONE',  ( -11.98357192835155338, -2.900346203988739102, 232.6627637660202481 ) ) ;
#11738=PLANE ( 'NONE',  #7771 ) ;
#11749=CARTESIAN_POINT ( 'NONE',  ( -0.03443693864400000637, -27.80022362959999782, 226.1000014189999945 ) ) ;
#11750=CARTESIAN_POINT ( 'NONE',  ( 24.07552309629999954, -13.90001137839999856, 223.9000014189999774 ) ) ;
#11757=CARTESIAN_POINT ( 'NONE',  ( -20.30396346370000060, 20.00000000000000000, 227.0000000000000000 ) ) ;
#11758=CARTESIAN_POINT ( 'NONE',  ( -27.77512470430000135, -2.247280056659999669E-11, 229.2930777930000090 ) ) ;
#11764=CARTESIAN_POINT ( 'NONE',  ( -24.11911872370000154, -15.18353100999999938, 224.6893563800000209 ) ) ;
#11782=CARTESIAN_POINT ( 'NONE',  ( 21.06251243579999866, -21.19733559970000414, 229.7625741969999922 ) ) ;
#11787=CARTESIAN_POINT ( 'NONE',  ( -1.070949874232112187, -27.77969728621822298, 225.2892653499953326 ) ) ;
#11791=CIRCLE ( 'NONE', #10800, 17.61822726820000184 ) ;
#11807=VERTEX_POINT ( 'NONE', #9246 ) ;
#11813=CIRCLE ( 'NONE', #29390, 26.80000000069999899 ) ;
#11814=FACE_OUTER_BOUND ( 'NONE', #23664, .T. ) ;
#11842=CARTESIAN_POINT ( 'NONE',  ( -23.55406855550000245, 16.04544956020000157, 222.0000000000000000 ) ) ;
#11848=ORIENTED_EDGE ( 'NONE', *, *, #25739, .T. ) ;
#11855=CARTESIAN_POINT ( 'NONE',  ( 24.53921759442506101, -13.06412590950472818, 225.5623281039913763 ) ) ;
#11857=CARTESIAN_POINT ( 'NONE',  ( 27.79999999999999716, 2.345590388590000174E-11, 222.0000000000000000 ) ) ;
#11858=CARTESIAN_POINT ( 'NONE',  ( 1.015231355570000105, -28.48218680760000154, 225.5064715119999903 ) ) ;
#11876=B_SPLINE_CURVE_WITH_KNOTS ( 'NONE', 5,
 ( #7219, #28765, #21393, #9257, #23918, #7373 ),
 .UNSPECIFIED., .F., .F.,
 ( 6, 6 ),
 ( -3.500000000000000000, 3.500000000000000000 ),
 .UNSPECIFIED. ) ;
#11891=CARTESIAN_POINT ( 'NONE',  ( 24.66410523950000311, -14.28055064019999953, 223.9000014189999774 ) ) ;
#11892=UNCERTAINTY_MEASURE_WITH_UNIT (LENGTH_MEASURE( 1.000000000000000082E-05 ), #10483, 'distance_accuracy_value', 'NONE');
#11900=CARTESIAN_POINT ( 'NONE',  ( 19.90436025690000221, 20.00000717710000231, 229.9507895630000007 ) ) ;
#11903=CARTESIAN_POINT ( 'NONE',  ( -1.063084826879999945, -27.77996807399999923, 225.3102023309999993 ) ) ;
#11904=CARTESIAN_POINT ( 'NONE',  ( 24.14759035961400713, -13.77518824758847416, 223.9000014190000059 ) ) ;
#11908=CARTESIAN_POINT ( 'NONE',  ( 3.378474373710000034, 11.51459555979999827, 232.0000000000000000 ) ) ;
#11911=ORIENTED_EDGE ( 'NONE', *, *, #12913, .T. ) ;
#11918=EDGE_LOOP ( 'NONE', ( #2700, #15578, #17892, #2222 ) ) ;
#11919=ORIENTED_EDGE ( 'NONE', *, *, #18840, .F. ) ;
#11932=CARTESIAN_POINT ( 'NONE',  ( -27.29823224869999976, -10.02941179569999974, 230.6577119970000069 ) ) ;
#11937=CARTESIAN_POINT ( 'NONE',  ( -0.1441937193057689637, -27.80022590917395675, 226.1000014190000229 ) ) ;
#11943=CARTESIAN_POINT ( 'NONE',  ( 27.79999999999999716, -2.355626804729999831E-11, 222.0000000000000000 ) ) ;
#11964=CARTESIAN_POINT ( 'NONE',  ( 23.62697774660000150, -14.64965012210000062, 225.6806946080000102 ) ) ;
#11995=CARTESIAN_POINT ( 'NONE',  ( -22.97554992469999746, 15.65135060219999907, 222.0000000000000000 ) ) ;
#12014=B_SPLINE_SURFACE_WITH_KNOTS ( 'NONE', 5, 1, ( 
 ( #23416, #11289 ),
 ( #1846, #11443 ),
 ( #26224, #23572 ),
 ( #30949, #8914 ),
 ( #18979, #26078 ),
 ( #9071, #6863 ),
 ( #11900, #21501 ),
 ( #2006, #4517 ),
 ( #28586, #18516 ),
 ( #28118, #31102 ),
 ( #16312, #14115 ),
 ( #6556, #20893 ),
 ( #21193, #13961 ),
 ( #7028, #6402 ),
 ( #25924, #4662 ) ),
 .UNSPECIFIED., .F., .F., .F.,
 ( 6, 3, 3, 3, 6 ),
 ( 2, 2 ),
 ( 0.000000000000000000, 0.5778133628420000223, 1.155626725680000133, 2.022346769939999955, 2.889066814210000000 ),
 ( -1.229628401229999994E-05, 0.7031504239110000221 ),
 .UNSPECIFIED. ) ;
#12016=CARTESIAN_POINT ( 'NONE',  ( 2.131628207279999844E-14, 1.421085471519999843E-14, 230.7531949689999919 ) ) ;
#12020=CARTESIAN_POINT ( 'NONE',  ( 24.48133297869999936, 13.22453720200000227, 222.0000000000000000 ) ) ;
#12029=LINE ( 'NONE', #28854, #24181 ) ;
#12034=EDGE_CURVE ( 'NONE', #25525, #10448, #29459, .T. ) ;
#12050=CARTESIAN_POINT ( 'NONE',  ( 24.68173674080000168, -14.25001227039999918, 223.9000014189999774 ) ) ;
#12051=CLOSED_SHELL ( 'NONE', ( #5601, #4146, #28101, #12223, #6987, #8853, #16354, #13809, #6800, #6163, #8749, #9855, #14426, #19383, #21000, #7587, #29058, #4451, #466, #16963, #20153, #20188, #30783, #5713, #5777, #17618, #22730, #5513, #3624, #4809, #11573, #14129, #9782, #28894, #17937, #12766, #3460, #2297, #23557, #10415, #4330, #560, #5579, #28237, #10633, #22157, #1228, #12489 ) ) ;
#12054=ORIENTED_EDGE ( 'NONE', *, *, #23476, .T. ) ;
#12056=CARTESIAN_POINT ( 'NONE',  ( 24.09856112909999837, -15.21545593799999985, 225.0000014190000002 ) ) ;
#12058=CARTESIAN_POINT ( 'NONE',  ( -4.751854023639999092, -11.13496319879999952, 231.9999989789999972 ) ) ;
#12059=CARTESIAN_POINT ( 'NONE',  ( -27.79999999999999716, -2.358050544769999872E-11, 226.2000000000000171 ) ) ;
#12065=CARTESIAN_POINT ( 'NONE',  ( -5.009717977351991536, -17.07423824983273875, 230.0306840897816016 ) ) ;
#12066=CARTESIAN_POINT ( 'NONE',  ( 4.374602741782418036, -11.28406995535170765, 232.0000002394077683 ) ) ;
#12072=CARTESIAN_POINT ( 'NONE',  ( 24.58943550720000104, -12.96928235400000062, 225.3105417090000060 ) ) ;
#12077=CARTESIAN_POINT ( 'NONE',  ( -23.41419870089999833, 16.84247076400000154, 229.0000000000000000 ) ) ;
#12083=CARTESIAN_POINT ( 'NONE',  ( 8.161936297539998719, -9.194081254939998615, 232.6627648150000027 ) ) ;
#12086=CARTESIAN_POINT ( 'NONE',  ( 28.35924375250000296, -2.486899575159999765E-14, 229.7625741969999922 ) ) ;
#12172=CARTESIAN_POINT ( 'NONE',  ( 24.82944511390000031, 13.78896019239999937, 229.1414195099999915 ) ) ;
#12173=CARTESIAN_POINT ( 'NONE',  ( 3.511461757819999807, 17.90077826259999938, 230.6999999999999886 ) ) ;
#12176=CARTESIAN_POINT ( 'NONE',  ( -1.100001419170000050, -27.77850706310000106, 225.0000014190000002 ) ) ;
#12187=DIRECTION ( 'NONE',  ( 0.000000000000000000, 0.000000000000000000, -1.000000000000000000 ) ) ;
#12204=CARTESIAN_POINT ( 'NONE',  ( -9.150307869779998882, 8.210980247390001097, 232.6627643349999914 ) ) ;
#12206=CARTESIAN_POINT ( 'NONE',  ( 19.80538212960000166, 19.50875458629999670, 229.0000000010000178 ) ) ;
#12221=ORIENTED_EDGE ( 'NONE', *, *, #8988, .F. ) ;
#12222=CARTESIAN_POINT ( 'NONE',  ( 25.20859211119999799, -13.29584934979999922, 225.3105417090000060 ) ) ;
#12223=ADVANCED_FACE ( 'NONE', ( #16609 ), #21951, .T. ) ;
#12230=DIRECTION ( 'NONE',  ( -0.2815395311429196301, -0.9595496299847262600, 0.000000000000000000 ) ) ;
#12238=CARTESIAN_POINT ( 'NONE',  ( 28.49999999970000175, -7.466149220240000162, 229.0000000000000000 ) ) ;
#12239=EDGE_LOOP ( 'NONE', ( #22182, #22219, #30284, #20713 ) ) ;
#12251=CARTESIAN_POINT ( 'NONE',  ( -18.50496050090000111, 20.74627092869999956, 229.0000000010000178 ) ) ;
#12257=ORIENTED_EDGE ( 'NONE', *, *, #3864, .F. ) ;
#12261=CARTESIAN_POINT ( 'NONE',  ( -26.80000000000000071, -8.704148513059999178E-14, 230.6999999999999886 ) ) ;
#12269=ORIENTED_EDGE ( 'NONE', *, *, #13979, .F. ) ;
#12272=CARTESIAN_POINT ( 'NONE',  ( -25.22658730140000216, -13.26242337740000110, 225.0000014190000002 ) ) ;
#12280=CARTESIAN_POINT ( 'NONE',  ( -23.50695179570000093, -14.84192241259999889, 225.0000014190000002 ) ) ;
#12293=CARTESIAN_POINT ( 'NONE',  ( 1.099998580829999906, -27.77839262550000043, 225.1040528159999781 ) ) ;
#12303=B_SPLINE_SURFACE_WITH_KNOTS ( 'NONE', 5, 1, ( 
 ( #8810, #30061 ),
 ( #11029, #28011 ),
 ( #8491, #11178 ),
 ( #22672, #22988 ),
 ( #6305, #1434 ),
 ( #25507, #16056 ),
 ( #18412, #1118 ),
 ( #6454, #29908 ),
 ( #2936, #9119 ),
 ( #289, #444 ),
 ( #14747, #1898 ),
 ( #14903, #28906 ),
 ( #19620, #9274 ),
 ( #9867, #4988 ),
 ( #28320, #5134 ) ),
 .UNSPECIFIED., .F., .F., .F.,
 ( 6, 3, 3, 3, 6 ),
 ( 2, 2 ),
 ( 0.000000000000000000, 0.5239049114000000618, 1.047809822800000124, 1.571714734199999963, 1.746349704670000058 ),
 ( -0.7000000000009999335, 2.557517976399999938E-06 ),
 .UNSPECIFIED. ) ;
#12316=CARTESIAN_POINT ( 'NONE',  ( -27.79999999999999716, -2.354383354940000152E-11, 222.0000000000000000 ) ) ;
#12335=CARTESIAN_POINT ( 'NONE',  ( 18.50497803210000214, 20.74625852780000201, 229.0000000010000178 ) ) ;
#12336=CARTESIAN_POINT ( 'NONE',  ( 5.114250173790000353, 17.43050733020000109, 230.6999999999999886 ) ) ;
#12350=ORIENTED_EDGE ( 'NONE', *, *, #15638, .F. ) ;
#12360=EDGE_LOOP ( 'NONE', ( #12416, #24936, #23483, #25309 ) ) ;
#12363=CARTESIAN_POINT ( 'NONE',  ( -2.808177005839999740, -11.72927066510000138, 231.9999989789999972 ) ) ;
#12386=ORIENTED_EDGE ( 'NONE', *, *, #22930, .F. ) ;
#12388=CARTESIAN_POINT ( 'NONE',  ( 28.50000000000000000, 1.065814103639999922E-14, 229.0000000000000000 ) ) ;
#12392=CARTESIAN_POINT ( 'NONE',  ( 7.780396774639999791, 9.519126025529999424, 232.6627648150000027 ) ) ;
#12408=CARTESIAN_POINT ( 'NONE',  ( -25.98395164609999952, 9.085482504939999870, 230.0000000000000000 ) ) ;
#12412=EDGE_CURVE ( 'NONE', #10989, #28017, #21557, .T. ) ;
#12416=ORIENTED_EDGE ( 'NONE', *, *, #16777, .F. ) ;
#12420=ORIENTED_EDGE ( 'NONE', *, *, #28962, .T. ) ;
#12434=CARTESIAN_POINT ( 'NONE',  ( 0.1441963505053185379, -27.80021098764100174, 226.1000014189999661 ) ) ;
#12437=CARTESIAN_POINT ( 'NONE',  ( 1.087695520339999833, -27.77888045939999984, 225.2081038119999903 ) ) ;
#12453=B_SPLINE_SURFACE_WITH_KNOTS ( 'NONE', 5, 1, ( 
 ( #19613, #10018 ),
 ( #8099, #3382 ),
 ( #22443, #889 ),
 ( #29670, #17692 ),
 ( #27307, #5749 ),
 ( #29816, #5897 ),
 ( #15502, #1513 ),
 ( #30620, #11258 ),
 ( #4020, #25584 ) ),
 .UNSPECIFIED., .F., .F., .F.,
 ( 6, 3, 6 ),
 ( 2, 2 ),
 ( 0.000000000000000000, 55.31395511720000258, 94.75474465359999954 ),
 ( -3.500000000000000000, 3.500000000000000000 ),
 .UNSPECIFIED. ) ;
#12480=CARTESIAN_POINT ( 'NONE',  ( 27.09307779329999732, 4.575104118570000544, 229.9751247039999953 ) ) ;
#12489=ADVANCED_FACE ( 'NONE', ( #30709 ), #10142, .T. ) ;
#12514=CARTESIAN_POINT ( 'NONE',  ( -4.885731407867048404, -11.07235429843764507, 232.0000000000045191 ) ) ;
#12519=SURFACE_STYLE_FILL_AREA ( #29354 ) ;
#12530=CARTESIAN_POINT ( 'NONE',  ( 24.39498713390000262, -13.33204241790000033, 225.9012973829999851 ) ) ;
#12547=CARTESIAN_POINT ( 'NONE',  ( 28.50000000000000000, 1.065814103639999922E-14, 229.0000000000000000 ) ) ;
#12558=EDGE_CURVE ( 'NONE', #24996, #23898, #24568, .T. ) ;
#12562=CARTESIAN_POINT ( 'NONE',  ( -17.87606967260930446, 20.00000012015441087, 230.7000000000000171 ) ) ;
#12563=CARTESIAN_POINT ( 'NONE',  ( -18.13790635940000229, 20.33475721459999974, 229.9172021029999939 ) ) ;
#12576=CARTESIAN_POINT ( 'NONE',  ( 24.55806919409999978, -14.46257963250000067, 226.0798541909999813 ) ) ;
#12594=CARTESIAN_POINT ( 'NONE',  ( 0.1059454459490000028, -28.50005195860000029, 226.0959520840000039 ) ) ;
#12597=APPLICATION_CONTEXT ( 'automotive_design' ) ;
#12611=CARTESIAN_POINT ( 'NONE',  ( 25.45460661299999927, 14.13620899649999885, 229.2404163060000144 ) ) ;
#12631=CARTESIAN_POINT ( 'NONE',  ( 26.72922997839999582, 9.361173623819999179, 229.4485730460000070 ) ) ;
#12632=CARTESIAN_POINT ( 'NONE',  ( -6.449395896350000434, -17.03876312330000076, 230.6999999999999886 ) ) ;
#12639=ORIENTED_EDGE ( 'NONE', *, *, #26804, .F. ) ;
#12666=CARTESIAN_POINT ( 'NONE',  ( -6.760206787919999627, 10.32311405969999996, 232.6627643349999914 ) ) ;
#12681=CARTESIAN_POINT ( 'NONE',  ( 24.11470756272141713, -15.18997277214834440, 224.7094697646042505 ) ) ;
#12686=B_SPLINE_CURVE_WITH_KNOTS ( 'NONE', 3,
 ( #13146, #6069, #14793, #24394, #17296, #23081, #25275, #30308, #29252, #27623, #24545, #10072, #2828, #15666, #10642, #3553, #11114, #1523, #3710, #18347, #20234, #20550, #13310, #20710, #3393, #22037, #1205, #8739, #20396, #1362, #10802, #8577, #17861, #1049, #488, #5909, #18178, #12998, #27782, #22610, #29828, #6227, #8266, #27467, #15511, #25118, #23232 ),
 .UNSPECIFIED., .F., .F.,
 ( 4, 2, 2, 2, 1, 1, 2, 2, 2, 2, 1, 1, 1, 2, 2, 2, 2, 1, 1, 1, 2, 2, 2, 2, 1, 2, 2, 4 ),
 ( 0.000000000000000000, 0.06250000000000112410, 0.1250000000000022482, 0.1875000000000033862, 0.2187499999999920897, 0.2343749999999864553, 0.2421874999999937272, 0.2500000000000009992, 0.3750000000001675882, 0.4375000000002438050, 0.4687500000002819411, 0.4843750000003009815, 0.4921875000003093081, 0.4960937500003123612, 0.5000000000003153033, 0.6250000000002886580, 0.6875000000002722267, 0.7187500000002626788, 0.7343750000002537970, 0.7421875000002519096, 0.7460937500002510214, 0.7500000000002501332, 0.8125000000001764144, 0.8437500000001433298, 0.8593750000001281197, 0.8671875000001204592, 0.8750000000001129097, 1.000000000000000000 ),
 .UNSPECIFIED. ) ;
#12693=CARTESIAN_POINT ( 'NONE',  ( -24.95819290936903911, -13.76152695242329216, 224.0343809112593476 ) ) ;
#12712=CARTESIAN_POINT ( 'NONE',  ( -19.95189713873627468, 20.00011557594780243, 229.8872997436589003 ) ) ;
#12719=ORIENTED_EDGE ( 'NONE', *, *, #3105, .F. ) ;
#12743=CARTESIAN_POINT ( 'NONE',  ( 2.131628207279999844E-14, 1.421085471519999843E-14, 231.6999999999999886 ) ) ;
#12747=CARTESIAN_POINT ( 'NONE',  ( 0.06886553587799999765, -27.80016486610000115, 226.0986540789999992 ) ) ;
#12751=CIRCLE ( 'NONE', #7716, 0.9999999999999981126 ) ;
#12754=CARTESIAN_POINT ( 'NONE',  ( 1.115119965759999943, -28.47834310740000063, 224.7918990269999995 ) ) ;
#12766=ADVANCED_FACE ( 'NONE', ( #30362 ), #26709, .F. ) ;
#12768=DIRECTION ( 'NONE',  ( 0.2665630446479613780, 0.9085064176298685013, -0.3218077568259533061 ) ) ;
#12789=CARTESIAN_POINT ( 'NONE',  ( -28.49999999979999998, 4.805538726630000923, 229.0000000000000000 ) ) ;
#12818=CARTESIAN_POINT ( 'NONE',  ( -13.70937177049999889, -27.52670431439999987, 229.4485705059999816 ) ) ;
#12825=UNCERTAINTY_MEASURE_WITH_UNIT (LENGTH_MEASURE( 1.000000000000000082E-05 ), #3705, 'distance_accuracy_value', 'NONE');
#12827=CARTESIAN_POINT ( 'NONE',  ( 18.62327035899999572, 19.80375215579999804, 229.9327584799999897 ) ) ;
#12841=FACE_OUTER_BOUND ( 'NONE', #8695, .T. ) ;
#12875=CARTESIAN_POINT ( 'NONE',  ( -19.67993405796693196, 20.00031463343183447, 230.1485629155865240 ) ) ;
#12876=CARTESIAN_POINT ( 'NONE',  ( -27.79999999999999716, -2.360422968200000068E-11, 229.0000000000000000 ) ) ;
#12887=VERTEX_POINT ( 'NONE', #29993 ) ;
#12905=CARTESIAN_POINT ( 'NONE',  ( -24.60699806910000120, -12.93667933180000063, 225.0000014190000002 ) ) ;
#12907=CARTESIAN_POINT ( 'NONE',  ( 0.1033071333810000048, -27.80005613150000343, 226.0959520840000039 ) ) ;
#12913=EDGE_CURVE ( 'NONE', #16560, #29420, #22765, .T. ) ;
#12918=CARTESIAN_POINT ( 'NONE',  ( -1.100001419170000050, -27.77850706310000106, 225.0000014190000002 ) ) ;
#12922=ORIENTED_EDGE ( 'NONE', *, *, #24808, .F. ) ;
#12934=CARTESIAN_POINT ( 'NONE',  ( 23.95489023949999918, -14.10735628980000023, 223.9201486480000085 ) ) ;
#12944=CARTESIAN_POINT ( 'NONE',  ( -27.35138618339999894, 9.563610239860000917, 229.7625741969999922 ) ) ;
#12946=EDGE_CURVE ( 'NONE', #29443, #21756, #27122, .T. ) ;
#12948=CARTESIAN_POINT ( 'NONE',  ( -5.114260856059999583, -17.43050419540000107, 230.6999999999999886 ) ) ;
#12961=ORIENTED_EDGE ( 'NONE', *, *, #12946, .T. ) ;
#12972=ORIENTED_EDGE ( 'NONE', *, *, #8126, .F. ) ;
#12976=CARTESIAN_POINT ( 'NONE',  ( 24.60666743799999878, -12.93650359530000138, 224.8958210039999983 ) ) ;
#12998=CARTESIAN_POINT ( 'NONE',  ( 18.43657771686843816, 20.00006074167432857, 230.6521199318109154 ) ) ;
#13042=CARTESIAN_POINT ( 'NONE',  ( 25.41516571979999739, -14.56554165020000013, 222.0000000000000000 ) ) ;
#13056=CARTESIAN_POINT ( 'NONE',  ( 20.30405755279999980, 20.00000000000000000, 229.0000000000000000 ) ) ;
#13075=VERTEX_POINT ( 'NONE', #23093 ) ;
#13085=CARTESIAN_POINT ( 'NONE',  ( 25.00924755590000004, -13.66774366000000107, 224.0987054560000047 ) ) ;
#13087=CARTESIAN_POINT ( 'NONE',  ( -26.07942841480000240, 9.118861015040000240, 230.6999999999999886 ) ) ;
#13093=CARTESIAN_POINT ( 'NONE',  ( 23.15117696689999960, -13.85641134509999972, 230.6999999999999886 ) ) ;
#13125=CARTESIAN_POINT ( 'NONE',  ( 24.58943550720000104, -12.96928235400000062, 224.6894611300000122 ) ) ;
#13127=CARTESIAN_POINT ( 'NONE',  ( 21.16705260759999874, -21.30254494060000070, 229.0000000000000000 ) ) ;
#13136=CARTESIAN_POINT ( 'NONE',  ( 19.80538173169999894, 19.50875421069999760, 227.5999999999999943 ) ) ;
#13138=B_SPLINE_CURVE_WITH_KNOTS ( 'NONE', 1,
 ( #6281, #13515 ),
 .UNSPECIFIED., .F., .F.,
 ( 2, 2 ),
 ( -2.556331299420000144E-06, 0.7000000000009999335 ),
 .UNSPECIFIED. ) ;
#13146=CARTESIAN_POINT ( 'NONE',  ( 20.30405755279999980, 20.00000000000000000, 229.0000000000000000 ) ) ;
#13167=CARTESIAN_POINT ( 'NONE',  ( 0.6677280494740716055, -27.79235729091802654, 224.1133967326756249 ) ) ;
#13171=CARTESIAN_POINT ( 'NONE',  ( -19.40755098202004802, 19.99999817177441841, 230.3222639546364405 ) ) ;
#13232=CARTESIAN_POINT ( 'NONE',  ( -0.07056952541309999272, -28.50017087330000010, 226.0986539140000104 ) ) ;
#13240=CARTESIAN_POINT ( 'NONE',  ( -26.80000000000000071, -7.731961996110000454E-14, 230.6999999999999886 ) ) ;
#13244=B_SPLINE_CURVE_WITH_KNOTS ( 'NONE', 1,
 ( #29270, #7711 ),
 .UNSPECIFIED., .F., .F.,
 ( 2, 2 ),
 ( -3.500000000000000000, 3.500000000000000000 ),
 .UNSPECIFIED. ) ;
#13246=CARTESIAN_POINT ( 'NONE',  ( -26.80000000000000071, -8.704148513059999178E-14, 230.6999999999999886 ) ) ;
#13269=CARTESIAN_POINT ( 'NONE',  ( 20.30405755279999980, 20.00000000000000000, 229.0000000000000000 ) ) ;
#13272=CARTESIAN_POINT ( 'NONE',  ( -27.79999999970000246, -10.21376199200000201, 229.0000000000000000 ) ) ;
#13286=CARTESIAN_POINT ( 'NONE',  ( 24.91921101730000032, -13.83103916679999834, 223.9972514410000031 ) ) ;
#13298=VERTEX_POINT ( 'NONE', #2767 ) ;
#13299=CARTESIAN_POINT ( 'NONE',  ( 26.95545381250000361, 8.667969360469999884, 222.0000000000000000 ) ) ;
#13303=EDGE_CURVE ( 'NONE', #979, #14446, #1466, .T. ) ;
#13309=ORIENTED_EDGE ( 'NONE', *, *, #23688, .T. ) ;
#13310=CARTESIAN_POINT ( 'NONE',  ( 19.42821516957057071, 19.99999712421914566, 230.3105388825946989 ) ) ;
#13329=CARTESIAN_POINT ( 'NONE',  ( -24.34159889609999894, -14.82483853620000147, 225.9014025209999943 ) ) ;
#13350=ORIENTED_EDGE ( 'NONE', *, *, #20365, .F. ) ;
#13355=CARTESIAN_POINT ( 'NONE',  ( 27.79999999999999716, -2.355626804729999831E-11, 222.0000000000000000 ) ) ;
#13360=CARTESIAN_POINT ( 'NONE',  ( 27.79999999990000248, 3.330083893049999855, 222.0000000000000000 ) ) ;
#13366=CARTESIAN_POINT ( 'NONE',  ( 1.099998580829999906, -27.77839262550000043, 224.8959500220000223 ) ) ;
#13368=CARTESIAN_POINT ( 'NONE',  ( -26.96951804470000269, 10.12763618690000023, 222.0000000000000000 ) ) ;
#13377=CARTESIAN_POINT ( 'NONE',  ( -133283.2432719999924, -454259.0741890000063, -160669.1380380000046 ) ) ;
#13384=VERTEX_POINT ( 'NONE', #26989 ) ;
#13388=ORIENTED_EDGE ( 'NONE', *, *, #19923, .F. ) ;
#13401=CARTESIAN_POINT ( 'NONE',  ( -23.94309786570000043, 13.28188914049999880, 230.6999999999999886 ) ) ;
#13402=CARTESIAN_POINT ( 'NONE',  ( 24.73445225629999911, -14.15837998019999944, 223.9040346120000038 ) ) ;
#13403=CARTESIAN_POINT ( 'NONE',  ( -22.55348085480000364, 18.07310466239999869, 229.0000000000000000 ) ) ;
#13407=CARTESIAN_POINT ( 'NONE',  ( -24.12155405280000053, -12.35224656769999996, 230.6999999999999886 ) ) ;
#13416=DIRECTION ( 'NONE',  ( 0.2665630446479613780, 0.9085064176298685013, -0.3218077568259533061 ) ) ;
#13428=CARTESIAN_POINT ( 'NONE',  ( -22.88601245399999939, -20.23007972099999563, 229.7313215430000071 ) ) ;
#13431=CARTESIAN_POINT ( 'NONE',  ( 1.099998580829999906, -27.77839262550000043, 225.0000014190000002 ) ) ;
#13432=CARTESIAN_POINT ( 'NONE',  ( -28.50002393070000295, -4.358072777779999203E-15, 222.0000000000000000 ) ) ;
#13441=CARTESIAN_POINT ( 'NONE',  ( 24.69936741169999905, -14.21947533890000059, 223.9000014189999774 ) ) ;
#13452=CARTESIAN_POINT ( 'NONE',  ( 26.95545381250000361, 8.667969382629999942, 224.8000000000000114 ) ) ;
#13461=CARTESIAN_POINT ( 'NONE',  ( -2.900346203986609694, 11.98357192835207741, 232.6627637660202481 ) ) ;
#13484=CARTESIAN_POINT ( 'NONE',  ( -24.25909092270000045, -14.95913241679999928, 225.7602679599999931 ) ) ;
#13503=ORIENTED_EDGE ( 'NONE', *, *, #30861, .F. ) ;
#13515=CARTESIAN_POINT ( 'NONE',  ( 3.550686850769999806E-05, -28.50022181210000127, 226.1000014189999945 ) ) ;
#13520=EDGE_CURVE ( 'NONE', #19036, #29420, #22274, .T. ) ;
#13541=VERTEX_POINT ( 'NONE', #9031 ) ;
#13549=CARTESIAN_POINT ( 'NONE',  ( -25.22658730140000216, -13.26242337740000110, 225.1042194559999814 ) ) ;
#13553=B_SPLINE_CURVE_WITH_KNOTS ( 'NONE', 1,
 ( #11995, #11842 ),
 .UNSPECIFIED., .F., .F.,
 ( 2, 2 ),
 ( -0.0003774847559270000114, 0.7000000095410000567 ),
 .UNSPECIFIED. ) ;
#13569=CARTESIAN_POINT ( 'NONE',  ( -24.34159889609999894, -14.82483853620000147, 225.9014025209999943 ) ) ;
#13570=CARTESIAN_POINT ( 'NONE',  ( 27.79999999980000069, -7.282770092329999834, 229.0000000000000000 ) ) ;
#13571=CARTESIAN_POINT ( 'NONE',  ( -19.80526744909999692, 19.50877353739999975, 229.0000000010000178 ) ) ;
#13573=ORIENTED_EDGE ( 'NONE', *, *, #532, .F. ) ;
#13576=ORIENTED_EDGE ( 'NONE', *, *, #28483, .F. ) ;
#13594=CARTESIAN_POINT ( 'NONE',  ( 27.79999999999999716, 2.356159711779999785E-11, 229.0000000000000000 ) ) ;
#13616=CARTESIAN_POINT ( 'NONE',  ( 19.80538173169999894, 19.50875421069999760, 222.0000000000000000 ) ) ;
#13617=EDGE_CURVE ( 'NONE', #5647, #13739, #5384, .T. ) ;
#13630=CARTESIAN_POINT ( 'NONE',  ( -18.15350094950000326, 19.92137095469999863, 229.9929676959999938 ) ) ;
#13644=CARTESIAN_POINT ( 'NONE',  ( -3.797468263909999919, 11.45463590949999855, 231.9999989789999972 ) ) ;
#13647=CARTESIAN_POINT ( 'NONE',  ( -24.68204616399999907, -14.25020164319999871, 226.1000014189999945 ) ) ;
#13648=CARTESIAN_POINT ( 'NONE',  ( -0.4820778520819999913, -28.49640832880000119, 226.0025182780000250 ) ) ;
#13676=CARTESIAN_POINT ( 'NONE',  ( 24.95644072989999884, -14.30264549059999979, 230.6577119970000069 ) ) ;
#13685=CARTESIAN_POINT ( 'NONE',  ( 1.127732790480000080, -28.47784299079999926, 225.0000014190000002 ) ) ;
#13701=ORIENTED_EDGE ( 'NONE', *, *, #2892, .T. ) ;
#13704=ORIENTED_EDGE ( 'NONE', *, *, #25344, .T. ) ;
#13714=CARTESIAN_POINT ( 'NONE',  ( -0.6685465368700000965, -28.49273882800000024, 225.9009104920000084 ) ) ;
#13722=CARTESIAN_POINT ( 'NONE',  ( -24.04140365350000152, -13.95971772459999904, 226.0986578890000089 ) ) ;
#13739=VERTEX_POINT ( 'NONE', #29929 ) ;
#13748=CARTESIAN_POINT ( 'NONE',  ( 25.41516571979999739, -14.56554165010000013, 229.1414211990000354 ) ) ;
#13760=CARTESIAN_POINT ( 'NONE',  ( -23.14178524820000149, 15.40497058279999898, 222.0000000000000000 ) ) ;
#13764=CARTESIAN_POINT ( 'NONE',  ( 27.24857305730000334, -4.377319704760001142E-12, 229.9172022069999741 ) ) ;
#13769=CARTESIAN_POINT ( 'NONE',  ( 27.79999999999999716, -2.355458807519999858E-11, 227.5999999999999943 ) ) ;
#13779=CARTESIAN_POINT ( 'NONE',  ( 3.441895497200000431, 11.73074891959999988, 232.6627635220000059 ) ) ;
#13783=CARTESIAN_POINT ( 'NONE',  ( -19.06889133170000150, 19.69230209619999883, 229.7995039799999972 ) ) ;
#13803=B_SPLINE_CURVE_WITH_KNOTS ( 'NONE', 1,
 ( #29001, #19411 ),
 .UNSPECIFIED., .F., .F.,
 ( 2, 2 ),
 ( 1.257340414754434539E-07, 0.7036780443879999680 ),
 .UNSPECIFIED. ) ;
#13804=CARTESIAN_POINT ( 'NONE',  ( -24.11911872370000154, -15.18353100999999938, 225.3106464589999973 ) ) ;
#13805=CARTESIAN_POINT ( 'NONE',  ( -1.127665019380000189, -28.47796022459999676, 225.0000014190000002 ) ) ;
#13807=CARTESIAN_POINT ( 'NONE',  ( 1.099998490678508523, -27.77839035186579508, 224.8530690857243428 ) ) ;
#13809=ADVANCED_FACE ( 'NONE', ( #20462 ), #12303, .T. ) ;
#13810=CARTESIAN_POINT ( 'NONE',  ( -20.30396346370000060, 20.00000000000000000, 227.3999999999999773 ) ) ;
#13817=CARTESIAN_POINT ( 'NONE',  ( -23.52673845780000050, -14.81058795080000046, 224.6893563800000209 ) ) ;
#13836=CARTESIAN_POINT ( 'NONE',  ( -13.87066093029999969, -27.85049402390000139, 230.2432540810000319 ) ) ;
#13858=B_SPLINE_CURVE_WITH_KNOTS ( 'NONE', 5,
 ( #22601, #1626, #1041, #11217, #20817, #18450 ),
 .UNSPECIFIED., .F., .F.,
 ( 6, 6 ),
 ( 0.000000000000000000, 18.03450582460000007 ),
 .UNSPECIFIED. ) ;
#13860=ORIENTED_EDGE ( 'NONE', *, *, #6289, .T. ) ;
#13865=CARTESIAN_POINT ( 'NONE',  ( 22.18615130530000101, 17.78888133539999927, 230.2432540810000319 ) ) ;
#13890=CARTESIAN_POINT ( 'NONE',  ( -18.32611925129999975, 20.54576746559999734, 229.7313256839999838 ) ) ;
#13896=B_SPLINE_CURVE_WITH_KNOTS ( 'NONE', 5,
 ( #30981, #14310, #28461, #9413, #14309, #26110, #14150, #16498, #28763, #25955, #30827, #23915, #2350, #21390, #2195 ),
 .UNSPECIFIED., .F., .F.,
 ( 6, 3, 3, 3, 6 ),
 ( 0.000000000000000000, 0.09999999999942736639, 0.3999999999977094656, 0.7000000000000000666, 1.000000000000000000 ),
 .UNSPECIFIED. ) ;
#13908=CARTESIAN_POINT ( 'NONE',  ( 27.79999999999999716, 2.355449169040000061E-11, 229.1414213560000235 ) ) ;
#13911=CARTESIAN_POINT ( 'NONE',  ( 28.50002393070000295, -9.769962616699999258E-14, 222.0000000000000000 ) ) ;
#13913=EDGE_LOOP ( 'NONE', ( #13704, #18249, #28787, #1134 ) ) ;
#13924=CARTESIAN_POINT ( 'NONE',  ( -27.16600648770000248, 9.122293387490000072, 222.0000000000000000 ) ) ;
#13942=ORIENTED_EDGE ( 'NONE', *, *, #2380, .F. ) ;
#13951=B_SPLINE_SURFACE_WITH_KNOTS ( 'NONE', 5, 1, ( 
 ( #19622, #24499 ),
 ( #2630, #9558 ),
 ( #26855, #24041 ),
 ( #12222, #12072 ),
 ( #26402, #21832 ),
 ( #5302, #19315 ),
 ( #15057, #14904 ),
 ( #2937, #12530 ),
 ( #21679, #292 ),
 ( #22138, #9869 ),
 ( #29060, #595 ),
 ( #10179, #19779 ),
 ( #29361, #7805 ),
 ( #17404, #27009 ),
 ( #5450, #30144 ) ),
 .UNSPECIFIED., .F., .F., .F.,
 ( 6, 3, 3, 3, 6 ),
 ( 2, 2 ),
 ( 0.000000000000000000, 0.5239010162220000266, 1.047802032450000143, 1.571703048660000102, 1.746336720740000015 ),
 ( -0.7000000000009999335, 2.556026448610000073E-06 ),
 .UNSPECIFIED. ) ;
#13959=DIRECTION ( 'NONE',  ( 1.000000000000000000, 0.000000000000000000, 0.000000000000000000 ) ) ;
#13961=CARTESIAN_POINT ( 'NONE',  ( 18.15340080560000047, 19.92139761430000178, 229.9929672670000116 ) ) ;
#13964=CARTESIAN_POINT ( 'NONE',  ( 1.871217339555081960, 11.95683682116809265, 232.0000000000053433 ) ) ;
#13965=CARTESIAN_POINT ( 'NONE',  ( -0.4702726639020000099, -27.79650200060000031, 226.0025182780000250 ) ) ;
#13969=CARTESIAN_POINT ( 'NONE',  ( -20.30396346370000060, 20.00000000000000000, 229.0000000000000000 ) ) ;
#13979=EDGE_CURVE ( 'NONE', #8755, #17736, #30053, .T. ) ;
#13980=CIRCLE ( 'NONE', #5432, 17.61822726820000184 ) ;
#13995=CARTESIAN_POINT ( 'NONE',  ( -28.50000000000000000, -3.552713678799999608E-15, 229.0000000000000000 ) ) ;
#14002=CARTESIAN_POINT ( 'NONE',  ( -24.26052213770000066, -13.57583965319999919, 223.9574921340000060 ) ) ;
#14015=DIRECTION ( 'NONE',  ( 0.000000000000000000, 0.000000000000000000, 1.000000000000000000 ) ) ;
#14024=CARTESIAN_POINT ( 'NONE',  ( -0.3831792618930000005, -28.49793954440000121, 223.9576764909999724 ) ) ;
#14034=CARTESIAN_POINT ( 'NONE',  ( -18.22457532099999611, 20.00000143240000128, 230.6880575950000036 ) ) ;
#14035=EDGE_CURVE ( 'NONE', #10061, #1204, #30846, .T. ) ;
#14045=CARTESIAN_POINT ( 'NONE',  ( 27.71720220739999974, 1.975538407690000167E-11, 229.4485730569999760 ) ) ;
#14050=FACE_OUTER_BOUND ( 'NONE', #13913, .T. ) ;
#14061=ORIENTED_EDGE ( 'NONE', *, *, #16777, .T. ) ;
#14067=CARTESIAN_POINT ( 'NONE',  ( 24.60666973300000038, -12.93650480179999995, 225.0000014190000002 ) ) ;
#14068=CARTESIAN_POINT ( 'NONE',  ( -18.90269220160000430, -21.67466784369999644, 222.0000000000000000 ) ) ;
#14094=AXIS2_PLACEMENT_3D ( 'NONE', #30119, #18147, #27751 ) ;
#14115=CARTESIAN_POINT ( 'NONE',  ( 18.62327035899999572, 19.80375215579999804, 229.9327584799999897 ) ) ;
#14118=CARTESIAN_POINT ( 'NONE',  ( -0.1033151399490000039, -27.80006701330000141, 226.0959516479999820 ) ) ;
#14120=CARTESIAN_POINT ( 'NONE',  ( 23.79608325624482745, -14.37377491939586349, 225.9639575250533881 ) ) ;
#14129=ADVANCED_FACE ( 'NONE', ( #26881 ), #9486, .T. ) ;
#14144=CARTESIAN_POINT ( 'NONE',  ( -5.408100974049999898, -10.71225608600000001, 231.9999991140000191 ) ) ;
#14148=CARTESIAN_POINT ( 'NONE',  ( 20.47082308819999952, -20.60185879389999997, 230.5592437530000041 ) ) ;
#14150=CARTESIAN_POINT ( 'NONE',  ( -24.43799431780000120, -14.66523353630000059, 223.9971937000000253 ) ) ;
#14175=CARTESIAN_POINT ( 'NONE',  ( -0.1058797546490000130, -28.50006311429999784, 223.9040511909999793 ) ) ;
#14184=AXIS2_PLACEMENT_3D ( 'NONE', #28728, #16310, #13959 ) ;
#14185=CARTESIAN_POINT ( 'NONE',  ( -20.30397143369999924, 20.00000785070000120, 229.0000000000000000 ) ) ;
#14208=ORIENTED_EDGE ( 'NONE', *, *, #4018, .F. ) ;
#14214=EDGE_CURVE ( 'NONE', #19036, #18684, #433, .T. ) ;
#14217=ORIENTED_EDGE ( 'NONE', *, *, #27010, .F. ) ;
#14218=CARTESIAN_POINT ( 'NONE',  ( 26.80000000000000071, -7.020799968500000432, 230.0000000000000000 ) ) ;
#14220=CARTESIAN_POINT ( 'NONE',  ( 24.40301908004844833, -13.31707607419617112, 225.8857039579157799 ) ) ;
#14221=CARTESIAN_POINT ( 'NONE',  ( 15.36964893400000065, -24.30838775939999863, 222.0000000000000000 ) ) ;
#14222=CARTESIAN_POINT ( 'NONE',  ( 0.8260714174469999671, -28.48835664879999996, 225.7596297540000023 ) ) ;
#14256=ORIENTED_EDGE ( 'NONE', *, *, #23476, .F. ) ;
#14262=CARTESIAN_POINT ( 'NONE',  ( 24.05832192679999793, -13.92979812329999945, 223.9000014189999774 ) ) ;
#14273=CARTESIAN_POINT ( 'NONE',  ( -25.27355175290000133, 12.75978488059999805, 224.8000000000000114 ) ) ;
#14301=CARTESIAN_POINT ( 'NONE',  ( 3.490170497419999851, -11.55197646250000076, 231.9999991140000191 ) ) ;
#14307=CARTESIAN_POINT ( 'NONE',  ( 24.50094951250000008, -14.04160150939999951, 230.6999999999999886 ) ) ;
#14309=CARTESIAN_POINT ( 'NONE',  ( -24.55841378230000061, -14.46270012129999927, 223.9201349020000009 ) ) ;
#14310=CARTESIAN_POINT ( 'NONE',  ( -24.66442003930000126, -14.28072947929999970, 223.9000014189999774 ) ) ;
#14314=CARTESIAN_POINT ( 'NONE',  ( 24.60666973300000038, -12.93650480179999995, 225.0000014190000002 ) ) ;
#14337=ORIENTED_EDGE ( 'NONE', *, *, #7121, .F. ) ;
#14342=CARTESIAN_POINT ( 'NONE',  ( 24.15870318760000046, -15.11998207899999969, 225.5069924249999929 ) ) ;
#14369=CARTESIAN_POINT ( 'NONE',  ( 25.00924755590000004, -13.66774365989999929, 225.9012973829999851 ) ) ;
#14387=B_SPLINE_CURVE_WITH_KNOTS ( 'NONE', 5,
 ( #30681, #6753, #9262, #9109, #25961, #14002, #2045, #11635, #21234, #18869, #23760, #24211, #14621, #21864, #9731 ),
 .UNSPECIFIED., .F., .F.,
 ( 6, 3, 3, 3, 6 ),
 ( 0.000000000000000000, 0.1000000000017179230, 0.4000000000011452173, 0.7000000000005726086, 1.000000000000000000 ),
 .UNSPECIFIED. ) ;
#14396=CARTESIAN_POINT ( 'NONE',  ( 27.53132593009999951, -1.219023768970000058E-11, 229.7313259299999686 ) ) ;
#14426=ADVANCED_FACE ( 'NONE', ( #6714 ), #29217, .F. ) ;
#14427=CARTESIAN_POINT ( 'NONE',  ( -27.79999999990000248, 4.328052761030000362, 229.0000000000000000 ) ) ;
#14443=CARTESIAN_POINT ( 'NONE',  ( 24.18127824746914811, -15.08370905573474374, 224.4394645126975547 ) ) ;
#14446=VERTEX_POINT ( 'NONE', #9546 ) ;
#14448=EDGE_LOOP ( 'NONE', ( #24891, #13309, #23622, #3904 ) ) ;
#14449=CARTESIAN_POINT ( 'NONE',  ( -27.63652367459999937, 8.874065151940001783, 229.0000000000000000 ) ) ;
#14460=CARTESIAN_POINT ( 'NONE',  ( 28.50000000000000000, -3.552713678799999608E-15, 229.2404163060000144 ) ) ;
#14466=CARTESIAN_POINT ( 'NONE',  ( -26.80000000000000071, 4.518892556970000030, 230.6999999999999886 ) ) ;
#14520=CARTESIAN_POINT ( 'NONE',  ( 21.81274943930000276, 17.27884304029999640, 223.9999999570000000 ) ) ;
#14551=CARTESIAN_POINT ( 'NONE',  ( 26.80907646719999704, 9.389153233529999198, 229.1414213529999984 ) ) ;
#14552=CARTESIAN_POINT ( 'NONE',  ( -18.02779420929999787, -3.032264855710000262, 230.6999999999999886 ) ) ;
#14562=CARTESIAN_POINT ( 'NONE',  ( 26.80000000069999899, 2.537275649180000148, 230.6999999999999886 ) ) ;
#14584=CARTESIAN_POINT ( 'NONE',  ( -4.775507269660000276, 11.08259804160000073, 231.9999989789999972 ) ) ;
#14585=CARTESIAN_POINT ( 'NONE',  ( -19.80526803549999926, 19.50877411520000138, 226.2000000000000171 ) ) ;
#14588=CARTESIAN_POINT ( 'NONE',  ( 24.59318164545437924, -12.96225840978618571, 224.7106956858033584 ) ) ;
#14594=CARTESIAN_POINT ( 'NONE',  ( 11.76275999642616199, 2.846903786951354931, 232.0000002394077399 ) ) ;
#14621=CARTESIAN_POINT ( 'NONE',  ( -24.60124998910000116, -12.94761260449999973, 224.7915656799999908 ) ) ;
#14628=CARTESIAN_POINT ( 'NONE',  ( -17.93345241809999990, 20.10553870999999759, 230.0000000000000000 ) ) ;
#14664=B_SPLINE_SURFACE_WITH_KNOTS ( 'NONE', 5, 1, ( 
 ( #27604, #17992 ),
 ( #25255, #12976 ),
 ( #15810, #10933 ),
 ( #1030, #13125 ),
 ( #29805, #17840 ),
 ( #16119, #6205 ),
 ( #30285, #3687 ),
 ( #22734, #27445 ),
 ( #13286, #8716 ),
 ( #20373, #22897 ),
 ( #6521, #25097 ),
 ( #4008, #15493 ),
 ( #1339, #8556 ),
 ( #13441, #18156 ),
 ( #3851, #23057 ) ),
 .UNSPECIFIED., .F., .F., .F.,
 ( 6, 3, 3, 3, 6 ),
 ( 2, 2 ),
 ( 0.000000000000000000, 0.5239010160280000994, 1.047802032050000109, 1.571703048080000054, 1.746336720089999961 ),
 ( -0.7000000000009999335, 2.556023926959999973E-06 ),
 .UNSPECIFIED. ) ;
#14696=CARTESIAN_POINT ( 'NONE',  ( 27.03927834839999989, 7.087470631950000488, 222.0000000000000000 ) ) ;
#14702=CARTESIAN_POINT ( 'NONE',  ( 18.44986304060000037, 20.68447005859999877, 229.4485727809999673 ) ) ;
#14722=B_SPLINE_SURFACE_WITH_KNOTS ( 'NONE', 5, 5, ( 
 ( #22745, #13769, #22910, #6059, #20698, #18168 ),
 ( #3696, #15654, #18334, #25108, #10787, #3862 ),
 ( #10943, #1350, #20539, #13452, #30136, #13299 ),
 ( #23221, #30297, #29975, #27613, #20385, #3540 ),
 ( #27771, #23070, #8727, #25265, #25433, #23390 ),
 ( #9044, #13136, #8884, #28239, #11104, #13616 ) ),
 .UNSPECIFIED., .F., .F., .F.,
 ( 6, 6 ),
 ( 6, 6 ),
 ( 0.000000000000000000, 21.89975014569999701 ),
 ( -3.500000000000000000, 3.500000000000000000 ),
 .UNSPECIFIED. ) ;
#14730=CARTESIAN_POINT ( 'NONE',  ( -6.635641388829999876, 10.13289756740000058, 231.9999989789999972 ) ) ;
#14732=CARTESIAN_POINT ( 'NONE',  ( -11.95683682116932545, 1.871217339555339976, 232.0000000000048601 ) ) ;
#14736=CARTESIAN_POINT ( 'NONE',  ( -26.80000000000000071, -7.283063041539999493E-14, 230.0000000000000000 ) ) ;
#14739=CARTESIAN_POINT ( 'NONE',  ( 23.50667118421176127, -14.84174322970506488, 225.1469793251989984 ) ) ;
#14742=CARTESIAN_POINT ( 'NONE',  ( 7.131609509308356465, -9.777910293739868308, 232.0000002394078535 ) ) ;
#14747=CARTESIAN_POINT ( 'NONE',  ( -24.80426825139999991, -14.03688870149999879, 223.9201349309999785 ) ) ;
#14776=CARTESIAN_POINT ( 'NONE',  ( -18.44984667599999639, 20.68448142150000280, 229.4485728150000057 ) ) ;
#14789=VERTEX_POINT ( 'NONE', #23215 ) ;
#14793=CARTESIAN_POINT ( 'NONE',  ( 20.29863583259346527, 20.00004025424676612, 229.1322715859966195 ) ) ;
#14830=CARTESIAN_POINT ( 'NONE',  ( -20.30396346370000060, 20.00000000000000000, 229.0000000000000000 ) ) ;
#14848=AXIS2_PLACEMENT_3D ( 'NONE', #12016, #7140, #16722 ) ;
#14863=CARTESIAN_POINT ( 'NONE',  ( -14.43445815169999946, 11.21795253560000027, 230.6999999999999886 ) ) ;
#14890=CARTESIAN_POINT ( 'NONE',  ( -2.860892586589999897, -11.94945454729999845, 232.6627643349999914 ) ) ;
#14892=CARTESIAN_POINT ( 'NONE',  ( -11.28407061768355568, -4.374602998566188283, 232.0000000000047464 ) ) ;
#14903=CARTESIAN_POINT ( 'NONE',  ( -24.73474822280000041, -14.15859640590000090, 223.9040321390000088 ) ) ;
#14904=CARTESIAN_POINT ( 'NONE',  ( 24.46818569879999927, -13.19686604630000026, 225.7601281139999969 ) ) ;
#14913=CARTESIAN_POINT ( 'NONE',  ( 1.776356839399999922E-14, 0.000000000000000000, 232.0000000000000000 ) ) ;
#14916=B_SPLINE_SURFACE_WITH_KNOTS ( 'NONE', 5, 1, ( 
 ( #30249, #22862 ),
 ( #6014, #15929 ),
 ( #8519, #1467 ),
 ( #29774, #8205 ),
 ( #30093, #27416 ),
 ( #30417, #27724 ),
 ( #10900, #11058 ),
 ( #13570, #5854 ),
 ( #15458, #25063 ) ),
 .UNSPECIFIED., .F., .F., .F.,
 ( 6, 3, 6 ),
 ( 2, 2 ),
 ( 0.000000000000000000, 53.95537973340000093, 92.42745556099998794 ),
 ( -3.500000000000000000, 3.500000000000000000 ),
 .UNSPECIFIED. ) ;
#14921=ORIENTED_EDGE ( 'NONE', *, *, #4802, .F. ) ;
#14928=CARTESIAN_POINT ( 'NONE',  ( 0.8694071509298356704, -27.78660432966791660, 224.3226506338012882 ) ) ;
#14933=CARTESIAN_POINT ( 'NONE',  ( -26.94142135619999934, 4.542738371190000457, 230.0000000000000000 ) ) ;
#14958=ORIENTED_EDGE ( 'NONE', *, *, #12558, .T. ) ;
#14966=CARTESIAN_POINT ( 'NONE',  ( -27.29823224880000154, -3.596834937749999341E-14, 230.6577119970000069 ) ) ;
#14987=CARTESIAN_POINT ( 'NONE',  ( 24.15098795939999832, 13.41224477779999980, 230.6999999999999886 ) ) ;
#14988=CARTESIAN_POINT ( 'NONE',  ( -28.49999999970000175, 7.466149641070000342, 229.0000000000000000 ) ) ;
#14999=CARTESIAN_POINT ( 'NONE',  ( 20.64716981389999972, -20.77933506589999979, 229.0000000020000073 ) ) ;
#15008=CARTESIAN_POINT ( 'NONE',  ( 27.79999999980000069, 4.694479351150000035, 229.1414213560000235 ) ) ;
#15039=ORIENTED_EDGE ( 'NONE', *, *, #27687, .T. ) ;
#15043=CARTESIAN_POINT ( 'NONE',  ( -5.304254813150000639E-10, 4.380584783799999468E-10, 230.0000000000000000 ) ) ;
#15044=CARTESIAN_POINT ( 'NONE',  ( -8.751033796364147577, -8.359833048263213939, 232.0000000000046043 ) ) ;
#15057=CARTESIAN_POINT ( 'NONE',  ( 25.08428924680000094, -13.52916357279999993, 225.7601281139999969 ) ) ;
#15060=ORIENTED_EDGE ( 'NONE', *, *, #29764, .T. ) ;
#15068=CARTESIAN_POINT ( 'NONE',  ( 12.06519527120000035, 0.2459946332740000075, 231.9999991140000191 ) ) ;
#15070=CARTESIAN_POINT ( 'NONE',  ( 28.45771199730000234, -1.776356839399999922E-14, 229.4982322489999831 ) ) ;
#15086=CARTESIAN_POINT ( 'NONE',  ( -26.94142135619999934, -1.741760412339999700E-13, 230.0000000000000000 ) ) ;
#15092=VERTEX_POINT ( 'NONE', #25985 ) ;
#15095=ORIENTED_EDGE ( 'NONE', *, *, #21187, .T. ) ;
#15120=CARTESIAN_POINT ( 'NONE',  ( 1.015231355539999880, -28.48218680760000154, 224.4935313260000100 ) ) ;
#15138=CARTESIAN_POINT ( 'NONE',  ( -19.80526803560000104, 19.50877411510000314, 228.5999999999999943 ) ) ;
#15145=DIRECTION ( 'NONE',  ( 1.000000000000000000, 0.000000000000000000, 0.000000000000000000 ) ) ;
#15150=CARTESIAN_POINT ( 'NONE',  ( -27.04041630560000087, -5.416379761039999262E-14, 230.6999999999999886 ) ) ;
#15153=CARTESIAN_POINT ( 'NONE',  ( 23.93626153989999850, 13.29299652659999964, 230.0000000000000000 ) ) ;
#15170=CARTESIAN_POINT ( 'NONE',  ( -22.39560851969999788, -19.79663304750000208, 230.0000000000000000 ) ) ;
#15181=VERTEX_POINT ( 'NONE', #7092 ) ;
#15185=CARTESIAN_POINT ( 'NONE',  ( 24.05832192679999793, -13.92979812329999945, 223.9000014189999774 ) ) ;
#15192=( NAMED_UNIT ( * ) PLANE_ANGLE_UNIT ( ) SI_UNIT ( $, .RADIAN. ) );
#15197=AXIS2_PLACEMENT_3D ( 'NONE', #19193, #21561, #5599 ) ;
#15213=CARTESIAN_POINT ( 'NONE',  ( -25.11462376325593837, -13.47330140865266834, 224.3201053094227859 ) ) ;
#15232=CARTESIAN_POINT ( 'NONE',  ( -27.53132593009999951, -1.221715529480000030E-11, 229.7313259299999686 ) ) ;
#15263=CARTESIAN_POINT ( 'NONE',  ( -24.59348680947261556, -12.96247199543289241, 225.2894582296841861 ) ) ;
#15271=CARTESIAN_POINT ( 'NONE',  ( 19.80538173989999962, 19.50875420239999869, 226.9999998930000231 ) ) ;
#15279=CARTESIAN_POINT ( 'NONE',  ( 4.960227444650000095, 16.90556345610000122, 230.0904314459999966 ) ) ;
#15307=CARTESIAN_POINT ( 'NONE',  ( -25.46187654339999895, 14.12439703449999939, 229.0000000000000000 ) ) ;
#15352=( NAMED_UNIT ( * ) SI_UNIT ( $, .STERADIAN. ) SOLID_ANGLE_UNIT ( ) );
#15388=CARTESIAN_POINT ( 'NONE',  ( -27.77512470430000135, -2.247288904110000173E-11, 229.2930777930000090 ) ) ;
#15397=ORIENTED_EDGE ( 'NONE', *, *, #20365, .T. ) ;
#15406=CARTESIAN_POINT ( 'NONE',  ( -21.17667619210000041, 18.05244527720000036, 225.0000000000000000 ) ) ;
#15415=DIRECTION ( 'NONE',  ( 0.000000000000000000, 0.000000000000000000, -1.000000000000000000 ) ) ;
#15456=CARTESIAN_POINT ( 'NONE',  ( -21.60246165930000117, 17.31101082549999859, 230.6577119970000069 ) ) ;
#15458=CARTESIAN_POINT ( 'NONE',  ( 27.79999999999999716, 2.355804440410000085E-11, 229.0000000000000000 ) ) ;
#15459=CARTESIAN_POINT ( 'NONE',  ( 14.43445127310000053, -11.21796138520000063, 230.6999999999999886 ) ) ;
#15483=CARTESIAN_POINT ( 'NONE',  ( -22.27803938659999972, -19.69272062099999943, 230.0000000000000000 ) ) ;
#15493=CARTESIAN_POINT ( 'NONE',  ( 24.12694114270000156, -13.81062811039999971, 223.9040346120000038 ) ) ;
#15495=CARTESIAN_POINT ( 'NONE',  ( -28.49999999959999641, -10.47094308429999998, 229.0000000000000000 ) ) ;
#15502=CARTESIAN_POINT ( 'NONE',  ( -26.05511412830000140, 14.93229958979999950, 229.0000000000000000 ) ) ;
#15511=CARTESIAN_POINT ( 'NONE',  ( 18.04539700001577529, 20.00000247597757408, 230.6997258737370942 ) ) ;
#15525=CARTESIAN_POINT ( 'NONE',  ( 27.29823224880000154, -5.927324070049999562E-14, 230.6577119970000069 ) ) ;
#15532=CARTESIAN_POINT ( 'NONE',  ( 0.1441797511781169050, -27.80021098851407402, 223.9000014190000627 ) ) ;
#15537=CARTESIAN_POINT ( 'NONE',  ( -20.03097513009040398, 19.99998374455136840, 229.7883118818511150 ) ) ;
#15567=CARTESIAN_POINT ( 'NONE',  ( 20.30405755279999980, 20.00000000000000000, 228.1999999569999886 ) ) ;
#15578=ORIENTED_EDGE ( 'NONE', *, *, #9715, .T. ) ;
#15581=ORIENTED_EDGE ( 'NONE', *, *, #28962, .F. ) ;
#15588=CARTESIAN_POINT ( 'NONE',  ( 27.56257419730000180, 3.635153433429999645E-14, 230.5592437530000041 ) ) ;
#15607=CARTESIAN_POINT ( 'NONE',  ( -22.44209336489999984, 17.98384493009999829, 229.7625741969999922 ) ) ;
#15613=CARTESIAN_POINT ( 'NONE',  ( 7.908773014210000341, 16.35323874420000223, 230.6999999999999886 ) ) ;
#15625=ORIENTED_EDGE ( 'NONE', *, *, #19160, .T. ) ;
#15638=EDGE_CURVE ( 'NONE', #453, #29484, #24431, .T. ) ;
#15646=CARTESIAN_POINT ( 'NONE',  ( 21.16705260770000052, -21.30254494060000070, 222.0000000000000000 ) ) ;
#15654=CARTESIAN_POINT ( 'NONE',  ( 27.79999999990000248, 4.333901782529999025, 227.5999999999999943 ) ) ;
#15666=CARTESIAN_POINT ( 'NONE',  ( 19.97801547478277584, 19.99997970718940010, 229.8634922149824149 ) ) ;
#15671=CARTESIAN_POINT ( 'NONE',  ( 21.16705260759999874, -21.30254494060000070, 229.0000000000000000 ) ) ;
#15681=CARTESIAN_POINT ( 'NONE',  ( 0.6688362735999796582, -27.79232735177769342, 225.8855372596424900 ) ) ;
#15706=B_SPLINE_CURVE_WITH_KNOTS ( 'NONE', 1,
 ( #16580, #16889 ),
 .UNSPECIFIED., .F., .F.,
 ( 2, 2 ),
 ( -0.0003775348956340000232, 0.7000000117410000167 ),
 .UNSPECIFIED. ) ;
#15713=CARTESIAN_POINT ( 'NONE',  ( 26.30490654700000164, 9.885210762690000763, 222.0000000000000000 ) ) ;
#15718=B_SPLINE_CURVE_WITH_KNOTS ( 'NONE', 5,
 ( #2489, #12077, #22143, #14449, #19164, #23902 ),
 .UNSPECIFIED., .F., .F.,
 ( 6, 6 ),
 ( 66.71879030859999204, 88.69760957229999576 ),
 .UNSPECIFIED. ) ;
#15725=CARTESIAN_POINT ( 'NONE',  ( 0.8260714173989999187, -28.48835664879999996, 224.2403730839999980 ) ) ;
#15730=EDGE_CURVE ( 'NONE', #29443, #23376, #16502, .T. ) ;
#15746=CARTESIAN_POINT ( 'NONE',  ( 17.83931934289999788, 20.00000000000000000, 230.6999999999999886 ) ) ;
#15748=CARTESIAN_POINT ( 'NONE',  ( -24.73474822280000041, -14.15859640590000090, 226.0959706989999916 ) ) ;
#15756=VECTOR ( 'NONE', #8328, 1000.000000000000114 ) ;
#15757=ORIENTED_EDGE ( 'NONE', *, *, #9844, .T. ) ;
#15765=CARTESIAN_POINT ( 'NONE',  ( -27.29823224880000154, -2.891194551069999571E-14, 230.6577119970000069 ) ) ;
#15770=CARTESIAN_POINT ( 'NONE',  ( 14.29505443750000104, -22.88289997660000097, 230.6999999999999886 ) ) ;
#15779=CARTESIAN_POINT ( 'NONE',  ( -25.22069443620000229, -13.27363204220000092, 225.2084371580000095 ) ) ;
#15795=CARTESIAN_POINT ( 'NONE',  ( -13.40068078979999910, -26.90685836619999804, 229.9751244090000171 ) ) ;
#15800=CARTESIAN_POINT ( 'NONE',  ( -28.49999999959999641, -10.47094308429999998, 229.0000000000000000 ) ) ;
#15810=CARTESIAN_POINT ( 'NONE',  ( 25.22036945370000183, -13.27344566769999901, 224.7916409239999780 ) ) ;
#15831=EDGE_CURVE ( 'NONE', #28749, #11807, #13896, .T. ) ;
#15840=CARTESIAN_POINT ( 'NONE',  ( -19.56389390649999882, 19.56881929660000097, 229.4993219170000032 ) ) ;
#15842=CARTESIAN_POINT ( 'NONE',  ( 24.07552037900000030, -13.90000980950000020, 226.1000014189999945 ) ) ;
#15850=ORIENTED_EDGE ( 'NONE', *, *, #1052, .F. ) ;
#15855=CARTESIAN_POINT ( 'NONE',  ( -24.48873108229999929, -14.58042505439999914, 226.0425106499999970 ) ) ;
#15890=CARTESIAN_POINT ( 'NONE',  ( 0.06886553588169999629, -27.80016486610000115, 223.9013487590000011 ) ) ;
#15908=CARTESIAN_POINT ( 'NONE',  ( 18.87722420200000073, 21.16361474609999860, 229.7625741969999922 ) ) ;
#15910=CARTESIAN_POINT ( 'NONE',  ( 7.908773014210000341, 16.35323874420000223, 230.6999999999999886 ) ) ;
#15929=CARTESIAN_POINT ( 'NONE',  ( -27.79999999970000246, -10.21376199200000201, 222.0000000000000000 ) ) ;
#15930=CARTESIAN_POINT ( 'NONE',  ( 8.621538427680000893, 16.00851259929999770, 230.6999999999999886 ) ) ;
#15952=CARTESIAN_POINT ( 'NONE',  ( 27.77512470430000135, 2.244249230899999945E-11, 229.2930777930000090 ) ) ;
#15956=CARTESIAN_POINT ( 'NONE',  ( -14.89627966379999968, -24.48058516850000288, 222.0000000000000000 ) ) ;
#15991=CARTESIAN_POINT ( 'NONE',  ( 23.83740787290000185, -14.30495753649999990, 226.0027499809999938 ) ) ;
#16022=PRODUCT_CONTEXT ( 'NONE', #20224, 'mechanical' ) ;
#16029=CARTESIAN_POINT ( 'NONE',  ( 5.445859840630000726, -10.81896303589999953, 231.9999991140000191 ) ) ;
#16049=B_SPLINE_CURVE_WITH_KNOTS ( 'NONE', 1,
 ( #6545, #30780 ),
 .UNSPECIFIED., .F., .F.,
 ( 2, 2 ),
 ( -0.7031504239110000221, -5.523706192445132501E-08 ),
 .UNSPECIFIED. ) ;
#16056=CARTESIAN_POINT ( 'NONE',  ( -24.50074272580000212, -13.13701158840000005, 224.3191686030000369 ) ) ;
#16066=CARTESIAN_POINT ( 'NONE',  ( 25.45460661299999927, 14.13620899630000061, 229.0000000000000000 ) ) ;
#16068=CARTESIAN_POINT ( 'NONE',  ( -24.19505510210000310, -13.69211658319999891, 226.0798679069999935 ) ) ;
#16095=CARTESIAN_POINT ( 'NONE',  ( -24.68204616399999907, -14.25020164319999871, 226.1000014189999945 ) ) ;
#16104=TOROIDAL_SURFACE ( 'NONE', #8044, 18.16530045470000232, 1.000000000000000000 ) ;
#16108=CARTESIAN_POINT ( 'NONE',  ( 5.096711188909999635, -30.05771175659999983, 229.9751249150000092 ) ) ;
#16110=CARTESIAN_POINT ( 'NONE',  ( -22.22795129429999861, -18.08627278310000008, 222.0000000000000000 ) ) ;
#16119=CARTESIAN_POINT ( 'NONE',  ( 25.11738521000000190, -13.46751580659999981, 224.3193205009999929 ) ) ;
#16133=FILL_AREA_STYLE_COLOUR ( '', #27362 ) ;
#16135=CARTESIAN_POINT ( 'NONE',  ( -10.52451944200266354, 6.422810504745973148, 232.6627637660202481 ) ) ;
#16155=EDGE_CURVE ( 'NONE', #4760, #17409, #8452, .T. ) ;
#16184=CARTESIAN_POINT ( 'NONE',  ( 9.431516900800000658E-09, 2.029448609160000227E-09, 230.0000000000000000 ) ) ;
#16188=CARTESIAN_POINT ( 'NONE',  ( -26.80000000000000071, -9.846360514330001479, 230.6999999999999886 ) ) ;
#16196=CARTESIAN_POINT ( 'NONE',  ( 1.115119965759999943, -28.47834310740000063, 224.7918990269999995 ) ) ;
#16199=B_SPLINE_SURFACE_WITH_KNOTS ( 'NONE', 5, 1, ( 
 ( #7551, #17141 ),
 ( #4572, #23782 ),
 ( #2223, #7090 ),
 ( #16678, #4733 ),
 ( #14342, #23941 ),
 ( #2378, #11964 ),
 ( #22, #18354 ),
 ( #2986, #7846 ),
 ( #17451, #15991 ),
 ( #27056, #10961 ),
 ( #12576, #22340 ),
 ( #8001, #11118 ),
 ( #25446, #27786 ),
 ( #6235, #5493 ),
 ( #10229, #15842 ) ),
 .UNSPECIFIED., .F., .F., .F.,
 ( 6, 3, 3, 3, 6 ),
 ( 2, 2 ),
 ( 0.000000000000000000, 0.5238999883160000426, 1.047799976630000129, 1.571699964950000084, 1.746333294390000068 ),
 ( -0.7000000000009999335, 2.555882182119999914E-06 ),
 .UNSPECIFIED. ) ;
#16205=B_SPLINE_CURVE_WITH_KNOTS ( 'NONE', 3,
 ( #22659, #25332, #27222, #29583, #1102, #29427, #3147, #17762, #27379, #15263, #5665, #12905 ),
 .UNSPECIFIED., .F., .F.,
 ( 4, 2, 2, 2, 2, 4 ),
 ( 0.000000000000000000, 0.2499999999999890643, 0.4999999999999781286, 0.6249999999999726885, 0.7499999999999671374, 1.000000000000000000 ),
 .UNSPECIFIED. ) ;
#16217=DIRECTION ( 'NONE',  ( 1.000000000000000000, 0.000000000000000000, 0.000000000000000000 ) ) ;
#16220=CARTESIAN_POINT ( 'NONE',  ( -25.27354923189999880, 12.75979636610000156, 229.0000000000000000 ) ) ;
#16226=CARTESIAN_POINT ( 'NONE',  ( -18.62349881349999947, 19.80369232029999793, 229.9327143820000003 ) ) ;
#16231=CARTESIAN_POINT ( 'NONE',  ( -17.83931601680000156, 20.00000000000000000, 230.7000111870000012 ) ) ;
#16235=CARTESIAN_POINT ( 'NONE',  ( 27.09307779339999911, 1.384329942100000039E-12, 229.9751247039999953 ) ) ;
#16261=CARTESIAN_POINT ( 'NONE',  ( -23.69219497580000322, -16.12132049240000242, 222.0000000000000000 ) ) ;
#16266=B_SPLINE_CURVE_WITH_KNOTS ( 'NONE', 3,
 ( #21670, #12065, #19304, #16776 ),
 .UNSPECIFIED., .F., .F.,
 ( 4, 4 ),
 ( 0.000000000000000000, 1.000000000000000000 ),
 .UNSPECIFIED. ) ;
#16272=CARTESIAN_POINT ( 'NONE',  ( 28.49999999979999998, -7.466149220249999274, 222.0000000000000000 ) ) ;
#16297=ORIENTED_EDGE ( 'NONE', *, *, #22578, .T. ) ;
#16310=DIRECTION ( 'NONE',  ( 0.000000000000000000, 0.000000000000000000, -1.000000000000000000 ) ) ;
#16312=CARTESIAN_POINT ( 'NONE',  ( 18.80688676539999804, 20.00000167889999858, 230.5857114979999949 ) ) ;
#16328=CARTESIAN_POINT ( 'NONE',  ( -23.56565371570000167, -14.74874063799999924, 224.4928788709999878 ) ) ;
#16329=ORIENTED_EDGE ( 'NONE', *, *, #28483, .T. ) ;
#16341=DIRECTION ( 'NONE',  ( 1.000000000000000000, 0.000000000000000000, 0.000000000000000000 ) ) ;
#16345=CARTESIAN_POINT ( 'NONE',  ( 5.353429552090000598, -31.57167681289999805, 229.4982322489999831 ) ) ;
#16354=ADVANCED_FACE ( 'NONE', ( #8238 ), #14664, .F. ) ;
#16375=CARTESIAN_POINT ( 'NONE',  ( 6.258113739069999681, 17.06910001600000015, 230.6999999999999886 ) ) ;
#16383=CARTESIAN_POINT ( 'NONE',  ( -19.36637386170000141, 20.00000465049999931, 230.3591670750000162 ) ) ;
#16396=FACE_OUTER_BOUND ( 'NONE', #18209, .T. ) ;
#16406=CARTESIAN_POINT ( 'NONE',  ( -19.80526803560000104, 19.50877411510000314, 227.0000000000000000 ) ) ;
#16416=CARTESIAN_POINT ( 'NONE',  ( 20.62869472290000061, -20.76074184889999685, 229.2930768649999891 ) ) ;
#16417=B_SPLINE_CURVE_WITH_KNOTS ( 'NONE', 5,
 ( #9969, #26795, #16577, #26185, #22235, #14999, #3641, #5697, #17647 ),
 .UNSPECIFIED., .F., .F.,
 ( 6, 3, 6 ),
 ( 0.000000000000000000, 53.20205529499999386, 91.13698440880000362 ),
 .UNSPECIFIED. ) ;
#16420=CARTESIAN_POINT ( 'NONE',  ( -0.9776373403070000023, -28.64054450000000074, 222.0000000000000000 ) ) ;
#16426=EDGE_CURVE ( 'NONE', #453, #4391, #15706, .T. ) ;
#16427=CARTESIAN_POINT ( 'NONE',  ( 4.456723356677985137, -11.49589600330395989, 232.6627637151898966 ) ) ;
#16452=CARTESIAN_POINT ( 'NONE',  ( -18.92356980859999993, 19.72862807099999927, 229.8505673220000176 ) ) ;
#16463=CARTESIAN_POINT ( 'NONE',  ( 24.43762869010000216, -14.66515636309999948, 226.0027499809999938 ) ) ;
#16465=CARTESIAN_POINT ( 'NONE',  ( -26.95773186790000153, 8.656139590820000507, 224.8000000000000114 ) ) ;
#16467=CARTESIAN_POINT ( 'NONE',  ( -0.3831792618880000556, -28.49793954440000121, 226.0423263479999889 ) ) ;
#16473=CARTESIAN_POINT ( 'NONE',  ( -27.71720220739999974, -1.978370540369999998E-11, 229.4485730569999760 ) ) ;
#16481=EDGE_LOOP ( 'NONE', ( #25317, #9810, #8294, #1744 ) ) ;
#16486=ORIENTED_EDGE ( 'NONE', *, *, #27010, .T. ) ;
#16496=CARTESIAN_POINT ( 'NONE',  ( 5.361384718760000112, -31.61859215129999967, 229.2404163060000144 ) ) ;
#16498=CARTESIAN_POINT ( 'NONE',  ( -24.34159889609999894, -14.82483853620000147, 224.0986003170000060 ) ) ;
#16502=B_SPLINE_CURVE_WITH_KNOTS ( 'NONE', 1,
 ( #25326, #8471 ),
 .UNSPECIFIED., .F., .F.,
 ( 2, 2 ),
 ( -2.556331278550000249E-06, 0.7000000000009999335 ),
 .UNSPECIFIED. ) ;
#16521=ORIENTED_EDGE ( 'NONE', *, *, #27513, .F. ) ;
#16557=FACE_OUTER_BOUND ( 'NONE', #4860, .T. ) ;
#16560=VERTEX_POINT ( 'NONE', #7601 ) ;
#16566=FACE_OUTER_BOUND ( 'NONE', #18724, .T. ) ;
#16569=CARTESIAN_POINT ( 'NONE',  ( 19.90445648569999904, -20.03186682420000153, 230.0000000000000000 ) ) ;
#16571=CARTESIAN_POINT ( 'NONE',  ( 27.16602884410000129, -9.122302432779999748, 222.0000000000000000 ) ) ;
#16577=CARTESIAN_POINT ( 'NONE',  ( -23.10935684530000245, -20.42749692129999772, 228.9999999990000106 ) ) ;
#16580=CARTESIAN_POINT ( 'NONE',  ( 22.97596755210000197, 15.65128466780000061, 222.0000000000000000 ) ) ;
#16582=CARTESIAN_POINT ( 'NONE',  ( -28.01992793520000191, 5.907563698139999708, 222.0000000000000000 ) ) ;
#16609=FACE_OUTER_BOUND ( 'NONE', #22689, .T. ) ;
#16616=CARTESIAN_POINT ( 'NONE',  ( 24.15870318760000046, -15.11998207899999969, 225.5069924249999929 ) ) ;
#16618=CARTESIAN_POINT ( 'NONE',  ( -22.83911268609999823, 16.42879705509999866, 227.5999999999999943 ) ) ;
#16620=CARTESIAN_POINT ( 'NONE',  ( 3.550686852090000366E-05, -28.50022181210000127, 226.1000014189999945 ) ) ;
#16632=CARTESIAN_POINT ( 'NONE',  ( -24.07583586439999834, -13.90018868249999962, 223.9000014189999774 ) ) ;
#16640=CARTESIAN_POINT ( 'NONE',  ( 20.30405755279999980, 20.00000000000000000, 229.0000000000000000 ) ) ;
#16648=CARTESIAN_POINT ( 'NONE',  ( -22.27803938659999972, -19.69272062099999943, 230.6999999999999886 ) ) ;
#16660=EDGE_CURVE ( 'NONE', #13541, #17736, #19860, .T. ) ;
#16678=CARTESIAN_POINT ( 'NONE',  ( 24.11883219139999923, -15.18335225210000061, 225.3105549429999996 ) ) ;
#16686=CARTESIAN_POINT ( 'NONE',  ( -20.15234898259999952, 20.00000753509999996, 229.6283026800000187 ) ) ;
#16695=DIRECTION ( 'NONE',  ( 0.2815395311429196301, 0.9595496299847262600, 0.000000000000000000 ) ) ;
#16708=B_SPLINE_CURVE_WITH_KNOTS ( 'NONE', 5,
 ( #28768, #24068, #3736, #26575, #6904, #7065 ),
 .UNSPECIFIED., .F., .F.,
 ( 6, 6 ),
 ( -7.118285296629999870, 0.000000000000000000 ),
 .UNSPECIFIED. ) ;
#16716=CARTESIAN_POINT ( 'NONE',  ( 24.60328987762038366, -12.94293973087761707, 225.1457708194568852 ) ) ;
#16718=CARTESIAN_POINT ( 'NONE',  ( 0.2462945485050000161, -28.49939181889999773, 226.0797949779999954 ) ) ;
#16722=DIRECTION ( 'NONE',  ( 1.000000000000000000, 0.000000000000000000, 0.000000000000000000 ) ) ;
#16727=CARTESIAN_POINT ( 'NONE',  ( -23.50695179570000093, -14.84192241259999889, 225.0000014190000002 ) ) ;
#16732=FACE_OUTER_BOUND ( 'NONE', #8303, .T. ) ;
#16748=ORIENTED_EDGE ( 'NONE', *, *, #23688, .F. ) ;
#16752=ORIENTED_EDGE ( 'NONE', *, *, #28936, .T. ) ;
#16755=B_SPLINE_CURVE_WITH_KNOTS ( 'NONE', 3,
 ( #1058, #910, #456, #12693, #19940, #29529, #15213, #17568, #29215, #26869, #27175, #17711 ),
 .UNSPECIFIED., .F., .F.,
 ( 4, 2, 2, 2, 2, 4 ),
 ( 0.000000000000000000, 0.2500000000000010547, 0.5000000000000021094, 0.6250000000000016653, 0.7500000000000011102, 1.000000000000000000 ),
 .UNSPECIFIED. ) ;
#16758=CARTESIAN_POINT ( 'NONE',  ( 20.30405755279999980, 20.00000000000000000, 226.9999998930000231 ) ) ;
#16760=CARTESIAN_POINT ( 'NONE',  ( 24.02382125689999981, -13.98923529139999999, 223.9040349389999847 ) ) ;
#16769=CARTESIAN_POINT ( 'NONE',  ( -26.95773186790000153, 8.656139628340000058, 222.0000000000000000 ) ) ;
#16772=CARTESIAN_POINT ( 'NONE',  ( -0.9902521520840001923, -27.78273347009999839, 225.5064930660000186 ) ) ;
#16773=CARTESIAN_POINT ( 'NONE',  ( -19.80526744909999692, 19.50877353739999975, 229.0000000010000178 ) ) ;
#16776=CARTESIAN_POINT ( 'NONE',  ( -5.114250173070000294, -17.43050732980000106, 230.0000000000000000 ) ) ;
#16777=EDGE_CURVE ( 'NONE', #16560, #10061, #24753, .T. ) ;
#16782=ORIENTED_EDGE ( 'NONE', *, *, #4064, .T. ) ;
#16808=CARTESIAN_POINT ( 'NONE',  ( -0.6677117243936687707, -27.79242653425564669, 225.8866279824144669 ) ) ;
#16809=CARTESIAN_POINT ( 'NONE',  ( -25.84755624059999946, 9.037785233809998431, 230.6999999999999886 ) ) ;
#16836=B_SPLINE_CURVE_WITH_KNOTS ( 'NONE', 3,
 ( #11750, #11904, #24028, #2470, #117, #17085, #9696, #19301, #4977, #14588, #21820, #19453 ),
 .UNSPECIFIED., .F., .F.,
 ( 4, 2, 2, 2, 2, 4 ),
 ( 0.000000000000000000, 0.2499999999999878431, 0.4999999999999756861, 0.6249999999999715783, 0.7499999999999674705, 1.000000000000000000 ),
 .UNSPECIFIED. ) ;
#16866=CARTESIAN_POINT ( 'NONE',  ( 22.97596238400000246, 15.65128114700000239, 222.0000000000000000 ) ) ;
#16875=ORIENTED_EDGE ( 'NONE', *, *, #10020, .F. ) ;
#16888=ORIENTED_EDGE ( 'NONE', *, *, #22187, .T. ) ;
#16889=CARTESIAN_POINT ( 'NONE',  ( 23.55447120710000064, 16.04539730700000177, 222.0000000000000000 ) ) ;
#16890=CARTESIAN_POINT ( 'NONE',  ( 25.09775673860000467, 13.55753231799999980, 222.0000000000000000 ) ) ;
#16894=CARTESIAN_POINT ( 'NONE',  ( 27.77512470410000134, 4.690278755559999624, 229.2930777930000090 ) ) ;
#16903=CARTESIAN_POINT ( 'NONE',  ( 17.83931934289999788, 20.00000000000000000, 230.6999999999999886 ) ) ;
#16915=CARTESIAN_POINT ( 'NONE',  ( 23.74337837439999888, -14.46065164910000078, 224.0987030360000176 ) ) ;
#16919=DIRECTION ( 'NONE',  ( -0.2815395311429196301, -0.9595496299847262600, 0.000000000000000000 ) ) ;
#16957=CARTESIAN_POINT ( 'NONE',  ( 12.29168530480000143, 0.2506124891389999720, 232.6627648150000027 ) ) ;
#16963=ADVANCED_FACE ( 'NONE', ( #17613 ), #28745, .F. ) ;
#16970=B_SPLINE_SURFACE_WITH_KNOTS ( 'NONE', 5, 5, ( 
 ( #23573, #23877, #14585, #24172, #23719, #7029 ),
 ( #2611, #16618, #4518, #26388, #18827, #7181 ),
 ( #28430, #2007, #4829, #14273, #2319, #31103 ),
 ( #21504, #21815, #19142, #16465, #270, #16769 ),
 ( #14427, #24025, #26079, #21354, #21663, #2467 ),
 ( #9851, #19450, #12059, #7488, #25925, #22858 ) ),
 .UNSPECIFIED., .F., .F., .F.,
 ( 6, 6 ),
 ( 6, 6 ),
 ( 66.71447726240000975, 88.61406016669999985 ),
 ( -3.500000000000000000, 3.500000000000000000 ),
 .UNSPECIFIED. ) ;
#16990=CARTESIAN_POINT ( 'NONE',  ( -0.3738033647229999645, -27.79799560440000050, 223.9576764909999724 ) ) ;
#17024=CARTESIAN_POINT ( 'NONE',  ( 20.50716141039999840, 18.79636021840000026, 225.9999999149999894 ) ) ;
#17031=CARTESIAN_POINT ( 'NONE',  ( -26.05511412830000140, 14.93229958979999950, 229.0000000000000000 ) ) ;
#17043=DIRECTION ( 'NONE',  ( 0.2815395311429195746, 0.9595496299847261490, 0.000000000000000000 ) ) ;
#17047=CARTESIAN_POINT ( 'NONE',  ( 24.10374060750000069, 15.23914466740000151, 222.0000000000000000 ) ) ;
#17050=B_SPLINE_CURVE_WITH_KNOTS ( 'NONE', 3,
 ( #7034, #31108, #7187, #14120, #4670, #280, #21200, #26689, #30798, #26541, #14739, #26233 ),
 .UNSPECIFIED., .F., .F.,
 ( 4, 2, 2, 2, 2, 4 ),
 ( 0.000000000000000000, 0.2500000000000126565, 0.5000000000000253131, 0.6250000000000296430, 0.7500000000000339728, 1.000000000000000000 ),
 .UNSPECIFIED. ) ;
#17053=CARTESIAN_POINT ( 'NONE',  ( 24.19803665890000133, 13.43835505600000069, 229.9751240860000223 ) ) ;
#17066=ORIENTED_EDGE ( 'NONE', *, *, #25344, .F. ) ;
#17070=B_SPLINE_SURFACE_WITH_KNOTS ( 'NONE', 5, 1, ( 
 ( #9159, #16866 ),
 ( #9478, #21603 ),
 ( #6966, #14520 ),
 ( #18921, #18762 ),
 ( #19081, #17024 ),
 ( #23968, #28363 ) ),
 .UNSPECIFIED., .F., .F., .F.,
 ( 6, 6 ),
 ( 2, 2 ),
 ( 0.000000000000000000, 7.118285296629999870 ),
 ( -0.7000000117410000167, 0.0003775348956340000232 ),
 .UNSPECIFIED. ) ;
#17081=CARTESIAN_POINT ( 'NONE',  ( 0.1347871022389999784, -12.22452263659999971, 232.6627643349999914 ) ) ;
#17085=CARTESIAN_POINT ( 'NONE',  ( 24.47668464858733373, -13.18089138023650975, 224.2673115778495685 ) ) ;
#17099=CARTESIAN_POINT ( 'NONE',  ( 24.60666973300000038, -12.93650480179999995, 225.0000014190000002 ) ) ;
#17128=CARTESIAN_POINT ( 'NONE',  ( -24.83650131330000121, 13.77747940689999950, 229.1414214410000056 ) ) ;
#17135=VERTEX_POINT ( 'NONE', #16773 ) ;
#17141=CARTESIAN_POINT ( 'NONE',  ( 23.50666810109999716, -14.84174128299999929, 225.0000014190000002 ) ) ;
#17149=CARTESIAN_POINT ( 'NONE',  ( -23.56894429787650935, -14.74331334052646980, 224.5038504355401017 ) ) ;
#17172=ORIENTED_EDGE ( 'NONE', *, *, #16426, .F. ) ;
#17199=CARTESIAN_POINT ( 'NONE',  ( 18.50497803200000035, 20.74625852820000205, 229.1414212620000228 ) ) ;
#17200=CARTESIAN_POINT ( 'NONE',  ( 1.854620136230000105, 18.18682247289999765, 230.6999999999999886 ) ) ;
#17223=B_SPLINE_SURFACE_WITH_KNOTS ( 'NONE', 5, 1, ( 
 ( #13685, #8799 ),
 ( #23288, #13366 ),
 ( #16196, #18709 ),
 ( #28466, #18557 ),
 ( #11168, #6597 ),
 ( #11015, #23454 ),
 ( #18401, #3933 ),
 ( #27839, #8635 ),
 ( #11329, #28308 ),
 ( #20763, #1732 ),
 ( #6903, #25493 ),
 ( #4396, #6291 ),
 ( #30370, #15890 ),
 ( #1884, #20926 ),
 ( #11483, #8958 ) ),
 .UNSPECIFIED., .F., .F., .F.,
 ( 6, 3, 3, 3, 6 ),
 ( 2, 2 ),
 ( 0.000000000000000000, 0.5239017170190000128, 1.047803434039999981, 1.571705151059999972, 1.746339056730000117 ),
 ( -0.7000000000009999335, 2.556331278550000249E-06 ),
 .UNSPECIFIED. ) ;
#17231=EDGE_CURVE ( 'NONE', #6392, #8755, #16836, .T. ) ;
#17232=CARTESIAN_POINT ( 'NONE',  ( -8.981701821569998856, 8.059682504060001307, 231.9999989789999972 ) ) ;
#17247=CARTESIAN_POINT ( 'NONE',  ( 24.33395417675687611, -14.83647238286172509, 224.1112557440231114 ) ) ;
#17251=EDGE_LOOP ( 'NONE', ( #13350, #4069, #14061, #16297 ) ) ;
#17253=ORIENTED_EDGE ( 'NONE', *, *, #29773, .F. ) ;
#17280=CARTESIAN_POINT ( 'NONE',  ( -26.81201737230000148, 9.375055877170000329, 229.1414213529999984 ) ) ;
#17286=ORIENTED_EDGE ( 'NONE', *, *, #22747, .T. ) ;
#17293=ORIENTED_EDGE ( 'NONE', *, *, #2701, .T. ) ;
#17296=CARTESIAN_POINT ( 'NONE',  ( 20.25970996295725968, 20.00000589292579534, 229.3324148076499114 ) ) ;
#17305=CARTESIAN_POINT ( 'NONE',  ( 5.114250173790000353, 17.43050733020000109, 230.6999999999999886 ) ) ;
#17318=CARTESIAN_POINT ( 'NONE',  ( 1.089891362629999971, -28.47934442809999922, 225.3101849020000031 ) ) ;
#17340=CARTESIAN_POINT ( 'NONE',  ( 26.80000000000000071, 3.019806626980000436E-14, 230.6999999999999886 ) ) ;
#17358=CARTESIAN_POINT ( 'NONE',  ( 21.43444001219999961, 17.18614031629999772, 229.9751245449999999 ) ) ;
#17365=PRODUCT_DEFINITION_FORMATION_WITH_SPECIFIED_SOURCE ( 'ANY', '', #1288, .NOT_KNOWN. ) ;
#17387=ORIENTED_EDGE ( 'NONE', *, *, #17755, .F. ) ;
#17392=CARTESIAN_POINT ( 'NONE',  ( -9.777910867663793582, -7.131609927916758629, 232.0000000000046612 ) ) ;
#17404=CARTESIAN_POINT ( 'NONE',  ( 24.69936741169999905, -14.21947533890000059, 226.1000014189999945 ) ) ;
#17409=VERTEX_POINT ( 'NONE', #19263 ) ;
#17415=CARTESIAN_POINT ( 'NONE',  ( 3.378474288950000126, 11.51459527090000101, 231.9999991140000191 ) ) ;
#17451=CARTESIAN_POINT ( 'NONE',  ( 24.43762869010000216, -14.66515636309999948, 226.0027499809999938 ) ) ;
#17462=CARTESIAN_POINT ( 'NONE',  ( 0.8746022926037627654, -27.78660248490213291, 225.6820510556075590 ) ) ;
#17489=CARTESIAN_POINT ( 'NONE',  ( 27.34838611700000044, 9.577833257040001769, 229.7625741969999922 ) ) ;
#17498=CARTESIAN_POINT ( 'NONE',  ( 24.15870318760000046, -15.11998207899999969, 224.4930104139999969 ) ) ;
#17503=CARTESIAN_POINT ( 'NONE',  ( -0.5615373373075090990, -28.49504780676721438, 224.0344865918038977 ) ) ;
#17510=CARTESIAN_POINT ( 'NONE',  ( 24.82944511390000031, 13.78896019219999936, 229.0000000000000000 ) ) ;
#17528=CARTESIAN_POINT ( 'NONE',  ( -13.25572673970000004, -26.61578565920000017, 230.0000000000000000 ) ) ;
#17536=CARTESIAN_POINT ( 'NONE',  ( 19.79266700209999996, 19.51190850369999907, 229.1494847489999813 ) ) ;
#17546=PRESENTATION_STYLE_ASSIGNMENT (( #738 ) ) ;
#17568=CARTESIAN_POINT ( 'NONE',  ( -25.15375632540583695, -13.40010330548238926, 224.4391897960165068 ) ) ;
#17580=CARTESIAN_POINT ( 'NONE',  ( -23.73488293864406629, -14.47501376178995258, 225.8859541126125237 ) ) ;
#17584=CARTESIAN_POINT ( 'NONE',  ( -18.21696450012034063, 20.00000023631326229, 230.6811166311184422 ) ) ;
#17598=ORIENTED_EDGE ( 'NONE', *, *, #22747, .F. ) ;
#17606=CARTESIAN_POINT ( 'NONE',  ( -19.80526803269999903, 19.50877411230000291, 227.0000000000000000 ) ) ;
#17613=FACE_OUTER_BOUND ( 'NONE', #26768, .T. ) ;
#17618=ADVANCED_FACE ( 'NONE', ( #10589, #6332, #23021, #18121 ), #14916, .T. ) ;
#17634=CARTESIAN_POINT ( 'NONE',  ( 28.04325408110000240, 2.413353885199999816E-14, 230.2432540810000319 ) ) ;
#17642=CARTESIAN_POINT ( 'NONE',  ( 24.11883219139999923, -15.18335225210000061, 224.6894478949999723 ) ) ;
#17647=CARTESIAN_POINT ( 'NONE',  ( 27.79999999999999716, 2.355804440410000085E-11, 229.0000000000000000 ) ) ;
#17650=CARTESIAN_POINT ( 'NONE',  ( -18.34692058799999970, 20.56908522310000009, 230.5592437530000041 ) ) ;
#17654=CARTESIAN_POINT ( 'NONE',  ( -21.27753346980000160, -16.59085281950000379, 230.6999999999999886 ) ) ;
#17682=FACE_BOUND ( 'NONE', #18741, .T. ) ;
#17684=CARTESIAN_POINT ( 'NONE',  ( 23.74337837439999888, -14.46065164910000078, 224.0987030360000176 ) ) ;
#17692=CARTESIAN_POINT ( 'NONE',  ( 14.09657531829999932, 28.30410039250000054, 222.0000000000000000 ) ) ;
#17709=PLANE ( 'NONE',  #19208 ) ;
#17711=CARTESIAN_POINT ( 'NONE',  ( -25.22658730140000216, -13.26242337740000110, 225.0000014190000002 ) ) ;
#17722=AXIS2_PLACEMENT_3D ( 'NONE', #2627, #14015, #29203 ) ;
#17731=CARTESIAN_POINT ( 'NONE',  ( -17.92761595767789728, 19.99992249444004244, 230.6995778483687616 ) ) ;
#17736=VERTEX_POINT ( 'NONE', #8998 ) ;
#17741=ORIENTED_EDGE ( 'NONE', *, *, #28936, .F. ) ;
#17755=EDGE_CURVE ( 'NONE', #11678, #28642, #28806, .T. ) ;
#17762=CARTESIAN_POINT ( 'NONE',  ( -24.53666176017020462, -13.06964705028265072, 225.5585889358212626 ) ) ;
#17765=CARTESIAN_POINT ( 'NONE',  ( -27.04041630560000087, -6.115355784250000757E-14, 230.6999999999999886 ) ) ;
#17785=CARTESIAN_POINT ( 'NONE',  ( 27.56257419730000180, 4.654386182180000553, 230.5592437530000041 ) ) ;
#17803=CARTESIAN_POINT ( 'NONE',  ( 24.68173674080000168, -14.25001227039999918, 223.9000014189999774 ) ) ;
#17804=FACE_OUTER_BOUND ( 'NONE', #26075, .T. ) ;
#17807=CARTESIAN_POINT ( 'NONE',  ( -19.80526803560000104, 19.50877411510000314, 227.8000000000000114 ) ) ;
#17815=EDGE_LOOP ( 'NONE', ( #14958, #27240, #16329, #26476 ) ) ;
#17824=ORIENTED_EDGE ( 'NONE', *, *, #15730, .F. ) ;
#17830=EDGE_CURVE ( 'NONE', #6392, #13541, #10823, .T. ) ;
#17840=CARTESIAN_POINT ( 'NONE',  ( 24.55535052759999814, -13.03386662210000146, 224.4930265309999982 ) ) ;
#17861=CARTESIAN_POINT ( 'NONE',  ( 18.66381637565261542, 19.99999441337020656, 230.6065604230005874 ) ) ;
#17871=CARTESIAN_POINT ( 'NONE',  ( -1.100001419170000050, -27.77850706310000106, 224.8959436220000043 ) ) ;
#17875=CARTESIAN_POINT ( 'NONE',  ( 26.80000000000000071, -6.394884621839999216E-14, 230.6999999999999886 ) ) ;
#17879=CARTESIAN_POINT ( 'NONE',  ( 19.80538173989999962, 19.50875420239999869, 227.3999999149999951 ) ) ;
#17886=CARTESIAN_POINT ( 'NONE',  ( -19.83759560044297388, 20.00030161953416297, 230.0085100852693358 ) ) ;
#17892=ORIENTED_EDGE ( 'NONE', *, *, #2380, .T. ) ;
#17903=CARTESIAN_POINT ( 'NONE',  ( 26.80000000069999899, -3.214342854470000215E-14, 230.0000000000000000 ) ) ;
#17937=ADVANCED_FACE ( 'NONE', ( #8167 ), #2849, .F. ) ;
#17949=CARTESIAN_POINT ( 'NONE',  ( -0.6817539855342577004, -28.49230123151905758, 224.1111716133609093 ) ) ;
#17952=CARTESIAN_POINT ( 'NONE',  ( 24.87112161019999945, -13.91739822849999975, 223.9575271749999672 ) ) ;
#17953=CARTESIAN_POINT ( 'NONE',  ( -21.81164872309999936, 17.47864169270000190, 230.5592437530000041 ) ) ;
#17957=CARTESIAN_POINT ( 'NONE',  ( 10.87630772340000185, -14.78838862870000170, 230.6999999999999886 ) ) ;
#17965=ORIENTED_EDGE ( 'NONE', *, *, #13617, .T. ) ;
#17990=CARTESIAN_POINT ( 'NONE',  ( 19.76610007289999871, 19.51851078889999869, 229.2246588520000046 ) ) ;
#17992=CARTESIAN_POINT ( 'NONE',  ( 24.60666743799999878, -12.93650359530000138, 225.0000014190000002 ) ) ;
#18030=CARTESIAN_POINT ( 'NONE',  ( 28.50000000000000000, 1.065814103639999922E-14, 229.0000000000000000 ) ) ;
#18050=EDGE_CURVE ( 'NONE', #24425, #17409, #4676, .T. ) ;
#18063=CARTESIAN_POINT ( 'NONE',  ( 5.229687933660000176, -30.84198039109999812, 222.0000000000000000 ) ) ;
#18090=ORIENTED_EDGE ( 'NONE', *, *, #70, .T. ) ;
#18096=CARTESIAN_POINT ( 'NONE',  ( -1.063084826889999945, -27.77996807399999923, 224.6898005070000011 ) ) ;
#18108=B_SPLINE_CURVE_WITH_KNOTS ( 'NONE', 5,
 ( #25046, #30229, #10719, #20320, #29919, #30076, #8042, #8503, #25197 ),
 .UNSPECIFIED., .F., .F.,
 ( 6, 3, 6 ),
 ( 0.000000000000000000, 55.31395627320000585, 94.75474476520000167 ),
 .UNSPECIFIED. ) ;
#18115=CARTESIAN_POINT ( 'NONE',  ( 25.20859211119999799, -13.29584934979999922, 224.6894611300000122 ) ) ;
#18116=CARTESIAN_POINT ( 'NONE',  ( -27.48714010850000022, 9.611077580710000845, 229.0000000000000000 ) ) ;
#18121=FACE_OUTER_BOUND ( 'NONE', #24192, .T. ) ;
#18122=CARTESIAN_POINT ( 'NONE',  ( 25.15543331629999813, -9.890973000660000736, 230.6999999999999886 ) ) ;
#18126=CARTESIAN_POINT ( 'NONE',  ( 20.30405755279999980, 20.00000000000000000, 227.7999999360000061 ) ) ;
#18131=CARTESIAN_POINT ( 'NONE',  ( -24.69967241520000201, -14.21967358789999913, 226.1000014189999945 ) ) ;
#18144=CARTESIAN_POINT ( 'NONE',  ( -23.10935684530000245, -20.42749692129999772, 228.9999999990000106 ) ) ;
#18147=DIRECTION ( 'NONE',  ( 0.000000000000000000, 0.000000000000000000, -1.000000000000000000 ) ) ;
#18156=CARTESIAN_POINT ( 'NONE',  ( 24.09271802129999784, -13.87022289859999979, 223.9000014189999774 ) ) ;
#18157=CARTESIAN_POINT ( 'NONE',  ( 24.09856112909999837, -15.21545593799999985, 225.0000014190000002 ) ) ;
#18166=ORIENTED_EDGE ( 'NONE', *, *, #12034, .F. ) ;
#18168=CARTESIAN_POINT ( 'NONE',  ( 27.79999999999999716, -2.355626804729999831E-11, 222.0000000000000000 ) ) ;
#18178=CARTESIAN_POINT ( 'NONE',  ( 18.53746668656496510, 20.00005358620013141, 230.6344766825556576 ) ) ;
#18179=ORIENTED_EDGE ( 'NONE', *, *, #17755, .T. ) ;
#18190=CARTESIAN_POINT ( 'NONE',  ( -0.9902521520970002378, -27.78273347009999839, 224.4935097720000101 ) ) ;
#18191=VERTEX_POINT ( 'NONE', #2510 ) ;
#18209=EDGE_LOOP ( 'NONE', ( #11848, #3988, #9484, #28302, #17965 ) ) ;
#18249=ORIENTED_EDGE ( 'NONE', *, *, #6762, .F. ) ;
#18255=CARTESIAN_POINT ( 'NONE',  ( 21.59673437689999886, 17.31628621529999990, 230.6577119970000069 ) ) ;
#18264=CARTESIAN_POINT ( 'NONE',  ( -1.115050571030000048, -28.47845913019999742, 225.2081166120000262 ) ) ;
#18276=CARTESIAN_POINT ( 'NONE',  ( -24.38821816920000174, 13.52880949539999911, 230.6577119970000069 ) ) ;
#18278=CARTESIAN_POINT ( 'NONE',  ( -23.62732472759999780, -14.64974168880000072, 225.6808321819999890 ) ) ;
#18282=CARTESIAN_POINT ( 'NONE',  ( -3.511472728539999810, -17.90077611009999714, 230.6999999999999886 ) ) ;
#18287=EDGE_LOOP ( 'NONE', ( #7271, #3614, #13576, #23437 ) ) ;
#18291=CARTESIAN_POINT ( 'NONE',  ( -24.80426825129999813, -14.03688870149999879, 226.0798679069999935 ) ) ;
#18309=CARTESIAN_POINT ( 'NONE',  ( 26.94142135619999934, 6.750155989720000084E-14, 230.0000000000000000 ) ) ;
#18334=CARTESIAN_POINT ( 'NONE',  ( 27.79999999990000248, 4.333901782529999025, 226.2000000000000171 ) ) ;
#18345=TOROIDAL_SURFACE ( 'NONE', #2283, 18.16530045470000232, 1.000000000000000000 ) ;
#18347=CARTESIAN_POINT ( 'NONE',  ( 19.47906472345739459, 20.00001843740129814, 230.2805668407570181 ) ) ;
#18354=CARTESIAN_POINT ( 'NONE',  ( 23.66291322330000213, -14.59162663150000050, 225.7601370010000039 ) ) ;
#18370=B_SPLINE_CURVE_WITH_KNOTS ( 'NONE', 1,
 ( #25931, #23426 ),
 .UNSPECIFIED., .F., .F.,
 ( 2, 2 ),
 ( -0.7000000000219999130, 5.329070518200751394E-15 ),
 .UNSPECIFIED. ) ;
#18390=CARTESIAN_POINT ( 'NONE',  ( 3.555688610909999881, -11.76883225949999989, 232.6627648150000027 ) ) ;
#18401=CARTESIAN_POINT ( 'NONE',  ( 0.8260714173989999187, -28.48835664879999996, 224.2403730839999980 ) ) ;
#18403=CARTESIAN_POINT ( 'NONE',  ( -28.49999999990000177, 3.410703877680000051, 222.0000000000000000 ) ) ;
#18412=CARTESIAN_POINT ( 'NONE',  ( -25.08454981450000076, -13.52946590090000178, 224.2397332909999932 ) ) ;
#18419=VERTEX_POINT ( 'NONE', #22426 ) ;
#18422=B_SPLINE_CURVE_WITH_KNOTS ( 'NONE', 5,
 ( #8206, #27266, #17807, #25219, #3975, #13571 ),
 .UNSPECIFIED., .F., .F.,
 ( 6, 6 ),
 ( -2.000000000000000000, 0.000000000000000000 ),
 .UNSPECIFIED. ) ;
#18440=CIRCLE ( 'NONE', #21463, 17.61822726820000184 ) ;
#18446=CARTESIAN_POINT ( 'NONE',  ( 20.30405755279999980, 20.00000000000000000, 227.3999999149999951 ) ) ;
#18450=CARTESIAN_POINT ( 'NONE',  ( 23.55447120710000064, 16.04539730700000177, 222.0000000000000000 ) ) ;
#18453=CARTESIAN_POINT ( 'NONE',  ( -24.71725143720000162, -14.18911829940000047, 226.0986578700000109 ) ) ;
#18468=CARTESIAN_POINT ( 'NONE',  ( -8.237618942580001047, -27.55517656820000028, 222.0000000000000000 ) ) ;
#18479=CARTESIAN_POINT ( 'NONE',  ( -26.49877110809999792, 8.898239018390000865, 222.0000000000000000 ) ) ;
#18504=CARTESIAN_POINT ( 'NONE',  ( -19.79257232079999795, 19.51192870039999860, 229.1494017060000203 ) ) ;
#18516=CARTESIAN_POINT ( 'NONE',  ( 19.06862361850000198, 19.69237242210000005, 229.7996270940000159 ) ) ;
#18531=CARTESIAN_POINT ( 'NONE',  ( -24.25909092259999866, -14.95913241689999928, 224.2397348780000073 ) ) ;
#18537=VERTEX_POINT ( 'NONE', #5501 ) ;
#18543=VECTOR ( 'NONE', #25287, 1000.000000000000000 ) ;
#18549=CARTESIAN_POINT ( 'NONE',  ( 26.05511440539999768, -14.93230011240000010, 229.0000000000000000 ) ) ;
#18557=CARTESIAN_POINT ( 'NONE',  ( 1.063086518139999992, -27.77985718819999761, 224.6898179359999972 ) ) ;
#18569=CARTESIAN_POINT ( 'NONE',  ( -27.79999999999999716, -2.354383354940000152E-11, 222.0000000000000000 ) ) ;
#18572=VERTEX_POINT ( 'NONE', #17305 ) ;
#18587=CARTESIAN_POINT ( 'NONE',  ( -17.83931601680000156, 20.00000000000000000, 230.7000111870000012 ) ) ;
#18603=CARTESIAN_POINT ( 'NONE',  ( -21.20818545079999851, 16.99505982179999819, 230.0000000000000000 ) ) ;
#18614=VERTEX_POINT ( 'NONE', #20282 ) ;
#18619=CARTESIAN_POINT ( 'NONE',  ( 5.214112608739999821, -30.75012229510000239, 229.4485748759999808 ) ) ;
#18633=CARTESIAN_POINT ( 'NONE',  ( -27.33171861409999792, 5.762471333930000661, 222.0000000000000000 ) ) ;
#18646=VECTOR ( 'NONE', #28192, 1000.000000000000114 ) ;
#18653=CARTESIAN_POINT ( 'NONE',  ( -19.76603762889999771, 19.51852293520000003, 229.2245375310000099 ) ) ;
#18666=CARTESIAN_POINT ( 'NONE',  ( 2.426970918150000323, 12.02853619149999886, 232.6627643349999914 ) ) ;
#18680=EDGE_CURVE ( 'NONE', #28330, #6498, #11876, .T. ) ;
#18681=CARTESIAN_POINT ( 'NONE',  ( -24.10559463919999956, -15.20494734660000091, 224.7915671760000009 ) ) ;
#18684=VERTEX_POINT ( 'NONE', #23757 ) ;
#18694=EDGE_CURVE ( 'NONE', #30938, #21756, #8116, .T. ) ;
#18695=B_SPLINE_CURVE_WITH_KNOTS ( 'NONE', 5,
 ( #30518, #28614, #7053, #28145, #30820, #1720 ),
 .UNSPECIFIED., .F., .F.,
 ( 6, 6 ),
 ( 0.000000000000000000, 1.000000000000000000 ),
 .UNSPECIFIED. ) ;
#18697=CARTESIAN_POINT ( 'NONE',  ( -5.208546124329999749, -11.06211866609999994, 232.6627648150000027 ) ) ;
#18701=CARTESIAN_POINT ( 'NONE',  ( -13.37464065170000005, -26.85454942340000173, 230.6999999999999886 ) ) ;
#18703=CARTESIAN_POINT ( 'NONE',  ( 24.84442124000000263, 12.90866478800000117, 222.0000000000000000 ) ) ;
#18709=CARTESIAN_POINT ( 'NONE',  ( 1.087695520339999833, -27.77888045939999984, 224.7918990269999995 ) ) ;
#18724=EDGE_LOOP ( 'NONE', ( #13860, #30150, #3950, #17253, #8334 ) ) ;
#18740=CARTESIAN_POINT ( 'NONE',  ( -19.65706407100000064, 20.00000595720000263, 230.1821686570000054 ) ) ;
#18741=EDGE_LOOP ( 'NONE', ( #6680, #19082, #25395, #10108 ) ) ;
#18748=CARTESIAN_POINT ( 'NONE',  ( -23.50695179570000093, -14.84192241259999889, 225.0000014190000002 ) ) ;
#18757=CARTESIAN_POINT ( 'NONE',  ( -27.71720220719999972, 4.673546953369999812, 229.4485730569999760 ) ) ;
#18762=CARTESIAN_POINT ( 'NONE',  ( 21.17691543559999801, 18.05241775060000009, 224.9999999359999947 ) ) ;
#18772=CARTESIAN_POINT ( 'NONE',  ( 20.64716981389999972, -20.77933506589999979, 229.0000000020000073 ) ) ;
#18781=CARTESIAN_POINT ( 'NONE',  ( 12.32633748798225071, -0.2818134555603850622, 232.6627636236952412 ) ) ;
#18786=CARTESIAN_POINT ( 'NONE',  ( 0.6686231747779999290, -28.49266848160000265, 225.9009072510000067 ) ) ;
#18792=ORIENTED_EDGE ( 'NONE', *, *, #4926, .T. ) ;
#18803=CARTESIAN_POINT ( 'NONE',  ( 0.2818134420171679588, 12.32633706535993312, 232.6627637660202197 ) ) ;
#18819=DIRECTION ( 'NONE',  ( 0.000000000000000000, 0.000000000000000000, 1.000000000000000000 ) ) ;
#18827=CARTESIAN_POINT ( 'NONE',  ( -22.83911268609999823, 16.42879705520000044, 223.3999999999999773 ) ) ;
#18836=CARTESIAN_POINT ( 'NONE',  ( -27.24857305730000334, -4.411353757410000576E-12, 229.9172022069999741 ) ) ;
#18840=EDGE_CURVE ( 'NONE', #55, #13075, #630, .T. ) ;
#18849=ORIENTED_EDGE ( 'NONE', *, *, #1024, .F. ) ;
#18861=CARTESIAN_POINT ( 'NONE',  ( -28.04325408079999704, -10.30313394320000064, 230.2432540810000319 ) ) ;
#18862=EDGE_LOOP ( 'NONE', ( #7548, #21784, #12639, #22135 ) ) ;
#18869=CARTESIAN_POINT ( 'NONE',  ( -24.50074272580000212, -13.13701158840000005, 224.3191686030000369 ) ) ;
#18892=CARTESIAN_POINT ( 'NONE',  ( -0.4702726640079999965, -27.79650200060000031, 223.9974845609999932 ) ) ;
#18906=CARTESIAN_POINT ( 'NONE',  ( -26.30711198659999894, 9.878896915450001259, 222.0000000000000000 ) ) ;
#18911=EDGE_CURVE ( 'NONE', #11807, #13075, #22738, .T. ) ;
#18914=ORIENTED_EDGE ( 'NONE', *, *, #18050, .F. ) ;
#18921=CARTESIAN_POINT ( 'NONE',  ( 21.71012070049999920, 18.50699920749999805, 224.9999999359999947 ) ) ;
#18930=CARTESIAN_POINT ( 'NONE',  ( 5.179147464839999770, -30.54390743120000096, 229.7313277700000071 ) ) ;
#18933=CARTESIAN_POINT ( 'NONE',  ( 23.46242932110000012, -15.37847435530000162, 222.0000000000000000 ) ) ;
#18944=CARTESIAN_POINT ( 'NONE',  ( -23.66805819309999848, 15.87731454680000098, 222.0000000000000000 ) ) ;
#18952=CARTESIAN_POINT ( 'NONE',  ( 27.79999999999999716, -2.355626804729999831E-11, 222.0000000000000000 ) ) ;
#18963=CARTESIAN_POINT ( 'NONE',  ( -11.49589586079802750, -4.456723305597296125, 232.6627637660202197 ) ) ;
#18979=CARTESIAN_POINT ( 'NONE',  ( 20.15227961529999945, 20.00000826590000003, 229.6286087310000141 ) ) ;
#18983=CARTESIAN_POINT ( 'NONE',  ( -1.127665019380000189, -28.47796022459999676, 225.1040592169999854 ) ) ;
#18990=CARTESIAN_POINT ( 'NONE',  ( -19.80526803560000104, 19.50877411510000314, 227.0000000000000000 ) ) ;
#18997=CARTESIAN_POINT ( 'NONE',  ( -24.05864279069999867, -13.92996648929999992, 223.9000014189999774 ) ) ;
#18999=EDGE_LOOP ( 'NONE', ( #17824, #12961, #2635, #8456 ) ) ;
#19011=CARTESIAN_POINT ( 'NONE',  ( 2.476301338670000352, -11.81090098049999959, 231.9999991140000191 ) ) ;
#19015=CARTESIAN_POINT ( 'NONE',  ( 21.16705260759999874, -21.30254494060000070, 229.0000000000000000 ) ) ;
#19036=VERTEX_POINT ( 'NONE', #12206 ) ;
#19043=B_SPLINE_SURFACE_WITH_KNOTS ( 'NONE', 5, 1, ( 
 ( #4199, #21045 ),
 ( #30645, #18666 ),
 ( #2158, #1691 ),
 ( #23876, #2317 ),
 ( #6710, #4047 ),
 ( #13644, #23248 ),
 ( #14584, #19141 ),
 ( #14730, #12666 ),
 ( #21662, #21972 ),
 ( #17232, #12204 ),
 ( #29186, #24326 ),
 ( #26836, #7788 ),
 ( #3068, #24171 ),
 ( #112, #9692 ),
 ( #24633, #9543 ),
 ( #7634, #19762 ),
 ( #2466, #22272 ),
 ( #5120, #2610 ),
 ( #28730, #24024 ),
 ( #22121, #21814 ),
 ( #2771, #426 ),
 ( #29040, #7487 ),
 ( #12058, #19296 ),
 ( #12363, #14890 ),
 ( #2918, #4973 ),
 ( #7179, #24482 ),
 ( #19449, #17081 ) ),
 .UNSPECIFIED., .F., .F., .F.,
 ( 6, 3, 3, 3, 3, 3, 3, 3, 6 ),
 ( 2, 2 ),
 ( 0.000000000000000000, 5.260060211419999909, 10.52012024700000126, 15.78018131380000000, 21.04024955639999916, 26.30030806260000276, 31.56036812210000164, 36.82042849589999634, 41.80426500389999944 ),
 ( -1.078245758850000184E-06, 0.7004350674429999923 ),
 .UNSPECIFIED. ) ;
#19044=ORIENTED_EDGE ( 'NONE', *, *, #29773, .T. ) ;
#19045=CARTESIAN_POINT ( 'NONE',  ( -1.419173372210000086E-06, -27.80022181310000207, 223.9000014189999774 ) ) ;
#19067=B_SPLINE_CURVE_WITH_KNOTS ( 'NONE', 5,
 ( #2927, #5126, #3230, #24334, #24641, #14736 ),
 .UNSPECIFIED., .F., .F.,
 ( 6, 6 ),
 ( 64.89339659379999148, 88.33140247330000250 ),
 .UNSPECIFIED. ) ;
#19081=CARTESIAN_POINT ( 'NONE',  ( 21.02350438529999721, 19.26967166389999875, 225.9999999149999894 ) ) ;
#19082=ORIENTED_EDGE ( 'NONE', *, *, #27687, .F. ) ;
#19084=EDGE_LOOP ( 'NONE', ( #21467, #12972, #28201, #4506 ) ) ;
#19094=CARTESIAN_POINT ( 'NONE',  ( 27.76736546530000282, -1.703869824139999878, 222.0000000000000000 ) ) ;
#19095=CARTESIAN_POINT ( 'NONE',  ( 0.8959394325450000807, -28.48619164239999790, 225.6801530179999986 ) ) ;
#19133=CARTESIAN_POINT ( 'NONE',  ( 1.776356839399999922E-14, 0.000000000000000000, 232.6627637660000119 ) ) ;
#19141=CARTESIAN_POINT ( 'NONE',  ( -4.865153911790000230, 11.29064247420000022, 232.6627643349999914 ) ) ;
#19142=CARTESIAN_POINT ( 'NONE',  ( -26.95773186790000153, 8.656139623419999651, 226.2000000000000171 ) ) ;
#19160=EDGE_CURVE ( 'NONE', #18191, #662, #23868, .T. ) ;
#19164=CARTESIAN_POINT ( 'NONE',  ( -28.49999999979999998, 4.437032521639999949, 229.0000000000000000 ) ) ;
#19174=CARTESIAN_POINT ( 'NONE',  ( 25.63755059829999894, -14.69299249370000204, 230.2432540810000319 ) ) ;
#19186=EDGE_CURVE ( 'NONE', #6392, #11688, #29086, .T. ) ;
#19190=ORIENTED_EDGE ( 'NONE', *, *, #13303, .T. ) ;
#19193=CARTESIAN_POINT ( 'NONE',  ( 0.6633312702179999798, 20.00000000000000000, 230.6999999999999886 ) ) ;
#19208=AXIS2_PLACEMENT_3D ( 'NONE', #29372, #3250, #2946 ) ;
#19227=ORIENTED_EDGE ( 'NONE', *, *, #12412, .T. ) ;
#19231=CARTESIAN_POINT ( 'NONE',  ( 24.87112161019999945, -13.91739822849999975, 226.0424756639999941 ) ) ;
#19257=EDGE_LOOP ( 'NONE', ( #29024, #11342, #29359, #12221 ) ) ;
#19259=FACE_OUTER_BOUND ( 'NONE', #3752, .T. ) ;
#19263=CARTESIAN_POINT ( 'NONE',  ( 7.908785388650001025, 16.35326433119999834, 230.0000000000000000 ) ) ;
#19265=CARTESIAN_POINT ( 'NONE',  ( -5.114260856059999583, -17.43050419540000107, 230.6999999999999886 ) ) ;
#19283=B_SPLINE_CURVE_WITH_KNOTS ( 'NONE', 3,
 ( #20254, #15532, #25137, #3573, #13167, #26885, #14928, #25462, #30006, #6716, #13807, #20572 ),
 .UNSPECIFIED., .F., .F.,
 ( 4, 2, 2, 2, 2, 4 ),
 ( 0.000000000000000000, 0.2500000000000104916, 0.5000000000000210942, 0.6250000000000264233, 0.7500000000000319744, 1.000000000000000000 ),
 .UNSPECIFIED. ) ;
#19284=B_SPLINE_CURVE_WITH_KNOTS ( 'NONE', 5,
 ( #24152, #14562, #21643, #26365, #23853, #7320, #91, #9670, #16903 ),
 .UNSPECIFIED., .F., .F.,
 ( 6, 3, 6 ),
 ( 0.000000000000000000, 18.05539734199999913, 32.16884876519999636 ),
 .UNSPECIFIED. ) ;
#19288=CARTESIAN_POINT ( 'NONE',  ( 24.09856112909999837, -15.21545593799999985, 225.0000014190000002 ) ) ;
#19289=FACE_OUTER_BOUND ( 'NONE', #11918, .T. ) ;
#19291=DIRECTION ( 'NONE',  ( 0.2815395311429191860, 0.9595496299847263710, 0.000000000000000000 ) ) ;
#19296=CARTESIAN_POINT ( 'NONE',  ( -4.841056642969999935, -11.34399063919999939, 232.6627643349999914 ) ) ;
#19301=CARTESIAN_POINT ( 'NONE',  ( 24.53642653790638661, -13.06930425982346300, 224.4416957644422155 ) ) ;
#19304=CARTESIAN_POINT ( 'NONE',  ( -5.061979081340524544, -17.25235576957286909, 230.0000000000073896 ) ) ;
#19305=B_SPLINE_SURFACE_WITH_KNOTS ( 'NONE', 5, 1, ( 
 ( #495, #17606 ),
 ( #20136, #27214 ),
 ( #5187, #15406 ),
 ( #5809, #8008 ),
 ( #19976, #29111 ),
 ( #22501, #951 ) ),
 .UNSPECIFIED., .F., .F., .F.,
 ( 6, 6 ),
 ( 2, 2 ),
 ( 0.000000000000000000, 7.118118795469999149 ),
 ( -0.7000000095410000567, 0.0003774847559270000114 ),
 .UNSPECIFIED. ) ;
#19306=CARTESIAN_POINT ( 'NONE',  ( 11.07235364852552628, -4.885731121097938612, 232.0000002394077114 ) ) ;
#19315=CARTESIAN_POINT ( 'NONE',  ( 24.50046877880000196, -13.13673243530000079, 225.6806823370000075 ) ) ;
#19328=CARTESIAN_POINT ( 'NONE',  ( 11.26446710299999943, -4.925455829439999711, 232.6627648150000027 ) ) ;
#19335=CARTESIAN_POINT ( 'NONE',  ( 11.26738311299999928, 4.321519186770000687, 231.9999991140000191 ) ) ;
#19339=B_SPLINE_SURFACE_WITH_KNOTS ( 'NONE', 5, 5, ( 
 ( #3816, #29771, #8203, #17650, #20489, #27414, #3490, #24751, #996 ),
 ( #25059, #30089, #15456, #17953, #8055, #15607, #20180, #6009, #13403 ),
 ( #8358, #1303, #18276, #8675, #10435, #10897, #27263, #3187, #15307 ),
 ( #5700, #13087, #27563, #25213, #25379, #12944, #8515, #23017, #18116 ),
 ( #3644, #27885, #5852, #27719, #6164, #10586, #22697, #843, #12789 ),
 ( #13240, #15150, #15765, #1463, #22857, #1140, #10733, #11055, #30244 ) ),
 .UNSPECIFIED., .F., .F., .F.,
 ( 6, 6 ),
 ( 6, 3, 6 ),
 ( 64.89339659389999326, 88.69760957229999576 ),
 ( 8.011061266649999624, 9.372199858680000162, 10.73333845069999981 ),
 .UNSPECIFIED. ) ;
#19371=CARTESIAN_POINT ( 'NONE',  ( -24.07583586439999834, -13.90018868249999962, 223.9000014189999774 ) ) ;
#19383=ADVANCED_FACE ( 'NONE', ( #28231 ), #22017, .T. ) ;
#19392=CARTESIAN_POINT ( 'NONE',  ( 24.71695093370000151, -14.18891100779999981, 226.0986570600000221 ) ) ;
#19404=B_SPLINE_CURVE_WITH_KNOTS ( 'NONE', 3,
 ( #1075, #12562, #17731, #10519, #29550, #8444, #7984, #29856, #17584, #22321, #30011, #27194, #22168, #27345, #5790, #10665, #5631, #20419, #20117, #20260, #5476, #10209, #24985, #24837, #19809, #8291, #3268, #27040, #13171, #29395, #7832, #24681, #12875, #17886, #5938, #12712, #22478, #1232, #15537, #25142, #3577, #22781, #1390, #30500, #30173, #22946, #28278, #6259 ),
 .UNSPECIFIED., .F., .F.,
 ( 4, 2, 2, 1, 2, 2, 2, 2, 1, 1, 2, 2, 2, 2, 1, 1, 1, 2, 2, 2, 2, 1, 1, 2, 2, 2, 2, 4 ),
 ( 0.000000000000000000, 0.06249999999991126542, 0.09374999999986689814, 0.1093749999998447076, 0.1171874999998356592, 0.1249999999998266109, 0.1874999999997725986, 0.2187499999997477573, 0.2343749999997364886, 0.2421874999997342404, 0.2460937499997351285, 0.2499999999997360445, 0.3749999999997508104, 0.4374999999997613020, 0.4687499999997650213, 0.4843749999997585820, 0.4921874999997553624, 0.4960937499997537525, 0.4999999999997520872, 0.6249999999996466160, 0.6874999999996009858, 0.7187499999995782263, 0.7343749999995679012, 0.7421874999995748956, 0.7499999999995818900, 0.8124999999996801447, 0.8749999999997782885, 1.000000000000000000 ),
 .UNSPECIFIED. ) ;
#19411=CARTESIAN_POINT ( 'NONE',  ( 27.79999999999999716, -2.355626804729999831E-11, 222.0000000000000000 ) ) ;
#19416=EDGE_CURVE ( 'NONE', #1204, #25525, #8065, .T. ) ;
#19419=CARTESIAN_POINT ( 'NONE',  ( 24.80722736699999942, 13.77662336740000093, 229.2930739560000006 ) ) ;
#19420=CARTESIAN_POINT ( 'NONE',  ( 0.1718132402369999812, 18.28024009670000183, 230.6999999999999886 ) ) ;
#19422=CARTESIAN_POINT ( 'NONE',  ( 19.80538212960000166, 19.50875458629999670, 229.0000000010000178 ) ) ;
#19430=ORIENTED_EDGE ( 'NONE', *, *, #28939, .F. ) ;
#19449=CARTESIAN_POINT ( 'NONE',  ( 0.1323034786299999988, -11.99927027549999892, 231.9999989789999972 ) ) ;
#19450=CARTESIAN_POINT ( 'NONE',  ( -27.79999999999999716, -2.359492241240000038E-11, 227.5999999999999943 ) ) ;
#19453=CARTESIAN_POINT ( 'NONE',  ( 24.60666973300000038, -12.93650480179999995, 225.0000014190000002 ) ) ;
#19467=VERTEX_POINT ( 'NONE', #27381 ) ;
#19468=CARTESIAN_POINT ( 'NONE',  ( 24.68173674080000168, -14.25001227039999918, 223.9000014189999774 ) ) ;
#19482=CARTESIAN_POINT ( 'NONE',  ( 10.85065064720000017, 5.281366379100000508, 231.9999991140000191 ) ) ;
#19496=CARTESIAN_POINT ( 'NONE',  ( 24.07552309629999954, -13.90001137839999856, 223.9000014189999774 ) ) ;
#19513=ORIENTED_EDGE ( 'NONE', *, *, #12034, .T. ) ;
#19525=LINE ( 'NONE', #29113, #18646 ) ;
#19554=ORIENTED_EDGE ( 'NONE', *, *, #19968, .T. ) ;
#19560=ORIENTED_EDGE ( 'NONE', *, *, #4018, .T. ) ;
#19576=CARTESIAN_POINT ( 'NONE',  ( 21.78117249990000204, 17.46412353909999737, 229.7313245359999883 ) ) ;
#19595=B_SPLINE_SURFACE_WITH_KNOTS ( 'NONE', 5, 5, ( 
 ( #26351, #4172, #4799, #13764, #14396, #83, #23996, #9661, #1820 ),
 ( #11409, #21012, #12480, #26806, #10439, #22094, #16894, #15008, #5550 ),
 ( #392, #10287, #29309, #7606, #24291, #12631, #551, #14551, #24143 ),
 ( #15153, #9977, #17053, #7756, #21782, #19731, #19419, #12172, #17510 ),
 ( #24453, #10132, #17358, #29009, #19576, #24755, #2887, #235, #3190 ),
 ( #22242, #26963, #2739, #20032, #5399, #14702, #24606, #17199, #12335 ) ),
 .UNSPECIFIED., .F., .F., .F.,
 ( 6, 6 ),
 ( 6, 3, 6 ),
 ( 0.000000000000000000, 23.43826350880000220 ),
 ( 8.011061266649999624, 8.811739692309998873, 9.612418117960000785 ),
 .UNSPECIFIED. ) ;
#19604=EDGE_CURVE ( 'NONE', #18684, #453, #16708, .T. ) ;
#19613=CARTESIAN_POINT ( 'NONE',  ( 28.50000000000000000, -1.776356839399999804E-15, 229.0000000000000000 ) ) ;
#19620=CARTESIAN_POINT ( 'NONE',  ( -24.71725143720000162, -14.18911829940000047, 223.9013449680000178 ) ) ;
#19622=CARTESIAN_POINT ( 'NONE',  ( 25.22625794089999829, -13.26224522399999906, 225.0000014190000002 ) ) ;
#19633=CARTESIAN_POINT ( 'NONE',  ( 9.816202962829999379, 7.095738861030000066, 231.9999991140000191 ) ) ;
#19655=CARTESIAN_POINT ( 'NONE',  ( -26.55289168650000065, 9.284439999669999111, 229.7313259189999712 ) ) ;
#19686=CARTESIAN_POINT ( 'NONE',  ( 1.127732790480000080, -28.47784299079999926, 225.1040528159999781 ) ) ;
#19700=CARTESIAN_POINT ( 'NONE',  ( -1.127665019380000189, -28.47796022459999676, 225.0000014190000002 ) ) ;
#19709=CARTESIAN_POINT ( 'NONE',  ( 27.29823224880000154, 3.129650177539999281E-14, 230.6577119970000069 ) ) ;
#19711=EDGE_CURVE ( 'NONE', #23898, #55, #8795, .T. ) ;
#19731=CARTESIAN_POINT ( 'NONE',  ( 24.75549318700000256, 13.74789704510000021, 229.4485677049999879 ) ) ;
#19732=CARTESIAN_POINT ( 'NONE',  ( -7.747012534260000471, -16.51919209409999922, 230.6999999999999886 ) ) ;
#19762=CARTESIAN_POINT ( 'NONE',  ( -12.18429361160000113, -1.640523776660000044, 232.6627643349999914 ) ) ;
#19779=CARTESIAN_POINT ( 'NONE',  ( 24.12694114270000156, -13.81062811039999971, 226.0959682270000144 ) ) ;
#19793=CARTESIAN_POINT ( 'NONE',  ( 11.05690487959999935, -4.834698001819999647, 231.9999991140000191 ) ) ;
#19801=CARTESIAN_POINT ( 'NONE',  ( -24.07583586439999834, -13.90018868249999962, 226.1000014189999945 ) ) ;
#19802=CARTESIAN_POINT ( 'NONE',  ( 2.131628207279999844E-14, 1.421085471519999843E-14, 231.6999999999999886 ) ) ;
#19809=CARTESIAN_POINT ( 'NONE',  ( -19.28886814869914801, 20.00013610278432807, 230.3850219899306921 ) ) ;
#19819=EDGE_CURVE ( 'NONE', #29443, #27611, #19283, .T. ) ;
#19838=CARTESIAN_POINT ( 'NONE',  ( -23.73536387410678117, -14.47423183427071258, 224.1131743014709627 ) ) ;
#19853=AXIS2_PLACEMENT_3D ( 'NONE', #19133, #7174, #16919 ) ;
#19860=B_SPLINE_CURVE_WITH_KNOTS ( 'NONE', 5,
 ( #17803, #3815, #1612, #13402, #27262, #17952, #3489, #13085, #3969, #5851, #6328, #18115, #994, #11202, #25058 ),
 .UNSPECIFIED., .F., .F.,
 ( 6, 3, 3, 3, 6 ),
 ( 0.000000000000000000, 0.1000000000005725753, 0.4000000000022904123, 0.6999999999994271915, 1.000000000000000000 ),
 .UNSPECIFIED. ) ;
#19869=CARTESIAN_POINT ( 'NONE',  ( 28.45771199710000232, 4.805544668949999654, 229.4982322489999831 ) ) ;
#19877=CARTESIAN_POINT ( 'NONE',  ( 24.04107748430000058, -13.95955969929999974, 223.9013459049999994 ) ) ;
#19904=CARTESIAN_POINT ( 'NONE',  ( -26.94142135619999934, 1.207922650790000128E-13, 230.0000000000000000 ) ) ;
#19918=CARTESIAN_POINT ( 'NONE',  ( 23.51325844009999955, -14.83130343779999905, 224.7916311099999973 ) ) ;
#19923=EDGE_CURVE ( 'NONE', #29481, #11688, #17050, .T. ) ;
#19932=ORIENTED_EDGE ( 'NONE', *, *, #5449, .T. ) ;
#19939=CARTESIAN_POINT ( 'NONE',  ( 28.50000000000000000, 1.065814103639999922E-14, 229.0000000000000000 ) ) ;
#19940=CARTESIAN_POINT ( 'NONE',  ( -25.01590170629258481, -13.65607539363486822, 224.1109849693008584 ) ) ;
#19968=EDGE_CURVE ( 'NONE', #26590, #18614, #16266, .T. ) ;
#19976=CARTESIAN_POINT ( 'NONE',  ( -22.97691952320000297, 16.89267704250000079, 223.0000000000000000 ) ) ;
#19988=CARTESIAN_POINT ( 'NONE',  ( -28.50000000000000000, -5.684341886079999373E-14, 229.0000000000000000 ) ) ;
#20019=CARTESIAN_POINT ( 'NONE',  ( 23.52644129050000288, -14.81042608839999808, 224.6894478949999723 ) ) ;
#20032=CARTESIAN_POINT ( 'NONE',  ( 18.13791608029999836, 20.33475167760000346, 229.9172020889999999 ) ) ;
#20051=EDGE_LOOP ( 'NONE', ( #5300, #25203, #9803, #18090 ) ) ;
#20088=CARTESIAN_POINT ( 'NONE',  ( -3.441895295100000141, -11.73074823080000151, 232.6627637660000119 ) ) ;
#20117=CARTESIAN_POINT ( 'NONE',  ( -18.63818496132067182, 19.99999332500478388, 230.6124940282188902 ) ) ;
#20136=CARTESIAN_POINT ( 'NONE',  ( -21.02335142420000125, 19.26967309480000168, 226.0000000000000000 ) ) ;
#20153=ADVANCED_FACE ( 'NONE', ( #12841 ), #12453, .F. ) ;
#20169=ORIENTED_EDGE ( 'NONE', *, *, #19416, .F. ) ;
#20173=CARTESIAN_POINT ( 'NONE',  ( 24.10531740749999940, -15.20475527630000023, 224.7916311099999973 ) ) ;
#20180=CARTESIAN_POINT ( 'NONE',  ( -22.52001623379999984, 18.04628797879999880, 229.4982322489999831 ) ) ;
#20183=CARTESIAN_POINT ( 'NONE',  ( 17.67198583300000081, 4.679695666559999800, 230.6999999999999886 ) ) ;
#20188=ADVANCED_FACE ( 'NONE', ( #6215 ), #14722, .T. ) ;
#20202=CARTESIAN_POINT ( 'NONE',  ( -27.53132593009999951, 1.223554590980000005E-11, 229.7313259299999686 ) ) ;
#20216=CARTESIAN_POINT ( 'NONE',  ( -14.09657507470000226, -28.30410041510000241, 229.0000000000000000 ) ) ;
#20224=APPLICATION_CONTEXT ( 'automotive_design' ) ;
#20234=CARTESIAN_POINT ( 'NONE',  ( 19.44955349022768942, 20.00000275008948591, 230.2981396233025464 ) ) ;
#20254=CARTESIAN_POINT ( 'NONE',  ( -1.419173372180000084E-06, -27.80022181310000207, 223.9000014189999774 ) ) ;
#20260=CARTESIAN_POINT ( 'NONE',  ( -18.63933997799378517, 19.99999301019102660, 230.6122333795804025 ) ) ;
#20261=CARTESIAN_POINT ( 'NONE',  ( -27.24857305730000334, -4.411440552420000435E-12, 229.9172022069999741 ) ) ;
#20264=EDGE_LOOP ( 'NONE', ( #16521, #17741, #23891, #19513 ) ) ;
#20279=CARTESIAN_POINT ( 'NONE',  ( -13.75032424529999986, -27.60893268180000248, 222.0000000000000000 ) ) ;
#20282=CARTESIAN_POINT ( 'NONE',  ( -5.114250173070000294, -17.43050732980000106, 230.0000000000000000 ) ) ;
#20288=CARTESIAN_POINT ( 'NONE',  ( 1.776356839399999922E-14, 0.000000000000000000, 232.0000000000000000 ) ) ;
#20296=CARTESIAN_POINT ( 'NONE',  ( 19.80538173989999962, 19.50875420239999869, 228.1999999569999886 ) ) ;
#20307=MECHANICAL_DESIGN_GEOMETRIC_PRESENTATION_REPRESENTATION('',(#10281),#3732);
#20313=CARTESIAN_POINT ( 'NONE',  ( 27.48412515190000249, 9.625371191550000205, 229.2404163060000144 ) ) ;
#20315=B_SPLINE_CURVE_WITH_KNOTS ( 'NONE', 1,
 ( #28557, #28853 ),
 .UNSPECIFIED., .F., .F.,
 ( 2, 2 ),
 ( -3.500000000000000000, 3.500000000000000000 ),
 .UNSPECIFIED. ) ;
#20317=MECHANICAL_DESIGN_GEOMETRIC_PRESENTATION_REPRESENTATION('',(#8240),#1733);
#20320=CARTESIAN_POINT ( 'NONE',  ( -14.09657507470000226, -28.30410041510000241, 222.0000000000000000 ) ) ;
#20325=CARTESIAN_POINT ( 'NONE',  ( -0.1058797546490000130, -28.50006311429999784, 226.0959516479999820 ) ) ;
#20336=CARTESIAN_POINT ( 'NONE',  ( 7.957576824819999395, -16.45835136280000199, 230.6999999999999886 ) ) ;
#20346=CARTESIAN_POINT ( 'NONE',  ( -25.08454981450000076, -13.52946590100000179, 225.7602695480000250 ) ) ;
#20349=ORIENTED_EDGE ( 'NONE', *, *, #19186, .F. ) ;
#20361=CARTESIAN_POINT ( 'NONE',  ( -27.24857305730000334, 4.416023102750000085E-12, 229.9172022069999741 ) ) ;
#20365=EDGE_CURVE ( 'NONE', #29420, #14789, #12029, .T. ) ;
#20373=CARTESIAN_POINT ( 'NONE',  ( 24.87112161019999945, -13.91739822849999975, 223.9575271749999672 ) ) ;
#20385=CARTESIAN_POINT ( 'NONE',  ( 25.26809617039999978, 12.77001320649999982, 223.3999999999999773 ) ) ;
#20393=CARTESIAN_POINT ( 'NONE',  ( -4.977446647723676953, -11.28020519024507706, 232.6627637660202197 ) ) ;
#20396=CARTESIAN_POINT ( 'NONE',  ( 18.83543878183406051, 20.00014484542172966, 230.5612148851877521 ) ) ;
#20402=CARTESIAN_POINT ( 'NONE',  ( -28.49999999959999641, -10.47094308429999998, 229.0000000000000000 ) ) ;
#20409=CARTESIAN_POINT ( 'NONE',  ( 28.04325408110000240, -4.147902640509999414E-14, 230.2432540810000319 ) ) ;
#20412=CARTESIAN_POINT ( 'NONE',  ( -24.66442003930000126, -14.28072947929999970, 226.1000014189999945 ) ) ;
#20419=CARTESIAN_POINT ( 'NONE',  ( -18.63196155432577328, 19.99999456996440017, 230.6139042306207898 ) ) ;
#20450=CARTESIAN_POINT ( 'NONE',  ( 0.03533597109940000286, -28.50021994999999819, 226.1000014189999945 ) ) ;
#20452=CARTESIAN_POINT ( 'NONE',  ( 20.30405755279999980, 20.00000000000000000, 228.5999999789999890 ) ) ;
#20454=CARTESIAN_POINT ( 'NONE',  ( 0.07063658732710000054, -28.50016343120000073, 223.9013487590000011 ) ) ;
#20462=FACE_OUTER_BOUND ( 'NONE', #5576, .T. ) ;
#20476=CIRCLE ( 'NONE', #6907, 26.79999999129999821 ) ;
#20489=CARTESIAN_POINT ( 'NONE',  ( -18.66688329739999830, 20.92780155480000204, 230.2432540810000319 ) ) ;
#20506=EDGE_LOOP ( 'NONE', ( #29068, #11919, #8609, #8140 ) ) ;
#20524=CARTESIAN_POINT ( 'NONE',  ( 19.68705805829999989, 19.53816415229999848, 229.3697640839999963 ) ) ;
#20539=CARTESIAN_POINT ( 'NONE',  ( 26.95545381250000361, 8.667969403609998125, 226.2000000000000171 ) ) ;
#20547=CARTESIAN_POINT ( 'NONE',  ( -6.422810504744110638, -10.52451944200381462, 232.6627637660203334 ) ) ;
#20550=CARTESIAN_POINT ( 'NONE',  ( 19.43676870293390735, 19.99999894348004759, 230.3055900836091325 ) ) ;
#20572=CARTESIAN_POINT ( 'NONE',  ( 1.099998580829999906, -27.77839262550000043, 225.0000014190000002 ) ) ;
#20594=CARTESIAN_POINT ( 'NONE',  ( 23.50667118420000179, -14.84174322970000048, 225.0000014190000002 ) ) ;
#20595=EDGE_CURVE ( 'NONE', #662, #26590, #19525, .T. ) ;
#20629=CARTESIAN_POINT ( 'NONE',  ( -1.127665019380000189, -28.47796022459999676, 224.8959436220000043 ) ) ;
#20632=CARTESIAN_POINT ( 'NONE',  ( -25.22069443620000229, -13.27363204220000092, 225.2084371580000095 ) ) ;
#20649=CARTESIAN_POINT ( 'NONE',  ( -24.43799431770000297, -14.66523353640000060, 226.0028091380000035 ) ) ;
#20652=CARTESIAN_POINT ( 'NONE',  ( 6.408200674649999762, -17.12117065109999814, 230.6999999999999886 ) ) ;
#20653=CARTESIAN_POINT ( 'NONE',  ( 7.670601361110000127, 15.86076312269999988, 230.0904314459999966 ) ) ;
#20677=CARTESIAN_POINT ( 'NONE',  ( 20.12213002960000097, -20.25093488000000264, 229.9751245540000184 ) ) ;
#20690=CARTESIAN_POINT ( 'NONE',  ( -25.64086162999999630, 11.13108295319999819, 222.0000000000000000 ) ) ;
#20698=CARTESIAN_POINT ( 'NONE',  ( 27.79999999999999716, -2.355675019179999893E-11, 223.3999999999999773 ) ) ;
#20705=SURFACE_STYLE_FILL_AREA ( #23227 ) ;
#20710=CARTESIAN_POINT ( 'NONE',  ( 19.42269931435233588, 19.99999652952873319, 230.3137021383872138 ) ) ;
#20713=ORIENTED_EDGE ( 'NONE', *, *, #15730, .T. ) ;
#20722=CARTESIAN_POINT ( 'NONE',  ( -1.419173372180000084E-06, -27.80022181310000207, 223.9000014189999774 ) ) ;
#20730=CARTESIAN_POINT ( 'NONE',  ( -24.15901410609999900, -15.12012600319999933, 225.5071239680000303 ) ) ;
#20743=EDGE_CURVE ( 'NONE', #6498, #18537, #23748, .T. ) ;
#20763=CARTESIAN_POINT ( 'NONE',  ( 0.3832430167609999772, -28.49789927060000139, 223.9576737099999946 ) ) ;
#20767=CARTESIAN_POINT ( 'NONE',  ( 19.80538173989999962, 19.50875420239999869, 227.7999999360000061 ) ) ;
#20789=CARTESIAN_POINT ( 'NONE',  ( -24.50074272580000212, -13.13701158850000006, 225.6808342349999918 ) ) ;
#20817=CARTESIAN_POINT ( 'NONE',  ( 25.46997661260000001, 13.23369636690000029, 222.0000000000000000 ) ) ;
#20836=CARTESIAN_POINT ( 'NONE',  ( 5.225008591809999992, -30.81438311299999810, 229.2930790960000138 ) ) ;
#20847=EDGE_CURVE ( 'NONE', #25525, #6418, #13244, .T. ) ;
#20867=AXIS2_PLACEMENT_3D ( 'NONE', #22586, #10315, #29961 ) ;
#20879=CARTESIAN_POINT ( 'NONE',  ( -19.68707896189999929, 19.53815547089999782, 229.3695869349999725 ) ) ;
#20886=DIRECTION ( 'NONE',  ( 0.000000000000000000, 0.000000000000000000, 1.000000000000000000 ) ) ;
#20893=CARTESIAN_POINT ( 'NONE',  ( 18.31087175629999919, 19.88197256460000162, 229.9783849850000195 ) ) ;
#20905=CARTESIAN_POINT ( 'NONE',  ( -24.55841378230000061, -14.46270012129999927, 223.9201349020000009 ) ) ;
#20920=CARTESIAN_POINT ( 'NONE',  ( -14.09657507470000226, -28.30410041510000241, 229.0000000000000000 ) ) ;
#20926=CARTESIAN_POINT ( 'NONE',  ( 0.03443198227100000008, -27.80021999669999744, 223.9000014189999774 ) ) ;
#20976=CARTESIAN_POINT ( 'NONE',  ( 22.97726876109999949, 16.89265187250000011, 222.9999999789999947 ) ) ;
#20980=ORIENTED_EDGE ( 'NONE', *, *, #21723, .T. ) ;
#20985=EDGE_LOOP ( 'NONE', ( #22908, #23935, #823, #199 ) ) ;
#21000=ADVANCED_FACE ( 'NONE', ( #4087 ), #17223, .F. ) ;
#21008=EDGE_CURVE ( 'NONE', #24996, #15092, #14387, .T. ) ;
#21012=CARTESIAN_POINT ( 'NONE',  ( 26.94142135619999934, 4.549494481000000867, 230.0000000000000000 ) ) ;
#21023=ORIENTED_EDGE ( 'NONE', *, *, #18680, .T. ) ;
#21045=CARTESIAN_POINT ( 'NONE',  ( 3.441895575009999764, 11.73074918480000051, 232.6627643349999914 ) ) ;
#21060=FACE_OUTER_BOUND ( 'NONE', #1241, .T. ) ;
#21074=DIRECTION ( 'NONE',  ( 0.000000000000000000, 0.000000000000000000, 1.000000000000000000 ) ) ;
#21078=CARTESIAN_POINT ( 'NONE',  ( 5.086809642800000475, -29.99929454970000009, 230.6999999999999886 ) ) ;
#21104=CARTESIAN_POINT ( 'NONE',  ( -1.115050571030000048, -28.47845913019999742, 224.7918862260000026 ) ) ;
#21106=CARTESIAN_POINT ( 'NONE',  ( -24.91946588839999777, -13.83134141909999926, 226.0028092389999870 ) ) ;
#21130=CARTESIAN_POINT ( 'NONE',  ( -27.09307779329999732, 4.568309977820000256, 229.9751247039999953 ) ) ;
#21145=CARTESIAN_POINT ( 'NONE',  ( 20.23761873489999985, -20.36716332730000190, 229.9172016509999992 ) ) ;
#21147=CARTESIAN_POINT ( 'NONE',  ( 3.916247328310000331, -28.49226594579999983, 222.0000000000000000 ) ) ;
#21158=CARTESIAN_POINT ( 'NONE',  ( -27.70209899609999837, 2.554093293449999802, 222.0000000000000000 ) ) ;
#21187=EDGE_CURVE ( 'NONE', #29481, #19467, #2342, .T. ) ;
#21190=ORIENTED_EDGE ( 'NONE', *, *, #5021, .T. ) ;
#21192=CARTESIAN_POINT ( 'NONE',  ( 1.099998580829999906, -27.77839262550000043, 225.0000014190000002 ) ) ;
#21193=CARTESIAN_POINT ( 'NONE',  ( 18.22444678769999982, 20.00000155620000086, 230.6880676309999956 ) ) ;
#21196=CARTESIAN_POINT ( 'NONE',  ( -2.846903954058784159, 11.76276068685684173, 232.0000000000052580 ) ) ;
#21198=CIRCLE ( 'NONE', #7618, 17.84349269770000035 ) ;
#21200=CARTESIAN_POINT ( 'NONE',  ( 23.62906798355282589, -14.64615088352157812, 225.6773072844200101 ) ) ;
#21203=CARTESIAN_POINT ( 'NONE',  ( -20.30396346370000060, 20.00000000000000000, 228.5999999999999943 ) ) ;
#21207=CARTESIAN_POINT ( 'NONE',  ( -24.43799431780000120, -14.66523353630000059, 223.9971937000000253 ) ) ;
#21224=CARTESIAN_POINT ( 'NONE',  ( -28.49999999959999641, -10.47094308429999998, 229.2404163060000144 ) ) ;
#21234=CARTESIAN_POINT ( 'NONE',  ( -24.46845037339999962, -13.19716075180000026, 224.2397332909999932 ) ) ;
#21272=CARTESIAN_POINT ( 'NONE',  ( -27.79999999999999716, -2.354383354940000152E-11, 222.0000000000000000 ) ) ;
#21273=CARTESIAN_POINT ( 'NONE',  ( -23.51354662350000169, -14.83147814589999847, 225.2084356629999888 ) ) ;
#21274=CARTESIAN_POINT ( 'NONE',  ( 27.77512470430000135, 2.244123299190000168E-11, 229.2930777930000090 ) ) ;
#21279=AXIS2_PLACEMENT_3D ( 'NONE', #23763, #30684, #6759 ) ;
#21281=VERTEX_POINT ( 'NONE', #4363 ) ;
#21283=CARTESIAN_POINT ( 'NONE',  ( -28.50000000000000000, -5.684341886079999373E-14, 229.0000000000000000 ) ) ;
#21299=CARTESIAN_POINT ( 'NONE',  ( 27.79999999980000069, -7.282770092329999834, 229.1414213560000235 ) ) ;
#21302=CARTESIAN_POINT ( 'NONE',  ( 24.14762151235643728, -13.77513428986648059, 226.1000014190000513 ) ) ;
#21303=CARTESIAN_POINT ( 'NONE',  ( 27.33171840929999874, -5.762472401450000170, 222.0000000000000000 ) ) ;
#21304=CARTESIAN_POINT ( 'NONE',  ( 0.03533597109940000286, -28.50021994999999819, 226.1000014189999945 ) ) ;
#21313=CARTESIAN_POINT ( 'NONE',  ( -23.55406854719999998, 16.04544955540000117, 222.0000000000000000 ) ) ;
#21348=ORIENTED_EDGE ( 'NONE', *, *, #21781, .T. ) ;
#21354=CARTESIAN_POINT ( 'NONE',  ( -27.79999999990000248, 4.328052761030000362, 224.8000000000000114 ) ) ;
#21362=CARTESIAN_POINT ( 'NONE',  ( 11.28406995534932555, 4.374602741788584659, 232.0000002394077683 ) ) ;
#21368=CARTESIAN_POINT ( 'NONE',  ( -23.66327188690000227, -14.59170227459999936, 224.2397348780000073 ) ) ;
#21372=ORIENTED_EDGE ( 'NONE', *, *, #21740, .F. ) ;
#21379=FACE_OUTER_BOUND ( 'NONE', #1429, .T. ) ;
#21383=CARTESIAN_POINT ( 'NONE',  ( -1.705642473229999956, -12.17534878329999870, 232.6627648150000027 ) ) ;
#21387=CARTESIAN_POINT ( 'NONE',  ( 21.13564515570000069, -21.27093644839999698, 229.4982322489999831 ) ) ;
#21390=CARTESIAN_POINT ( 'NONE',  ( -24.09883371379999772, -15.21565466309999870, 224.8957841300000098 ) ) ;
#21393=CARTESIAN_POINT ( 'NONE',  ( -27.79999999999999716, -2.358036054649999912E-11, 226.2000000000000171 ) ) ;
#21427=CARTESIAN_POINT ( 'NONE',  ( -19.18334381879999739, 20.00000379799999806, 230.4459753579999983 ) ) ;
#21433=CARTESIAN_POINT ( 'NONE',  ( -22.97554992469999746, 15.65135060219999907, 222.0000000000000000 ) ) ;
#21458=CARTESIAN_POINT ( 'NONE',  ( 24.07552309629999954, -13.90001137829999855, 226.1000014189999945 ) ) ;
#21463=AXIS2_PLACEMENT_3D ( 'NONE', #28873, #12187, #24472 ) ;
#21465=DIRECTION ( 'NONE',  ( 0.000000000000000000, 0.000000000000000000, 1.000000000000000000 ) ) ;
#21467=ORIENTED_EDGE ( 'NONE', *, *, #1052, .T. ) ;
#21494=CARTESIAN_POINT ( 'NONE',  ( 24.64642659020000082, -14.31106159850000026, 223.9013459049999994 ) ) ;
#21501=CARTESIAN_POINT ( 'NONE',  ( 19.49298387170000169, 19.58648673140000440, 229.5592795560000070 ) ) ;
#21504=CARTESIAN_POINT ( 'NONE',  ( -26.95773186790000153, 8.656139628340000058, 229.0000000000000000 ) ) ;
#21529=EDGE_LOOP ( 'NONE', ( #7159, #17066, #12054, #18179 ) ) ;
#21535=MANIFOLD_SOLID_BREP ( 'PartBody', #12051 ) ;
#21536=CARTESIAN_POINT ( 'NONE',  ( 10.00047450490000145, 7.228941357680000124, 232.6627648150000027 ) ) ;
#21540=CARTESIAN_POINT ( 'NONE',  ( -28.35924375250000296, 0.000000000000000000, 229.7625741969999922 ) ) ;
#21545=CARTESIAN_POINT ( 'NONE',  ( -0.2820369105234935003, -27.79912531870053272, 226.0732182084217641 ) ) ;
#21546=CARTESIAN_POINT ( 'NONE',  ( -21.20818545079999851, 16.99505982179999819, 230.6999999999999886 ) ) ;
#21557=B_SPLINE_CURVE_WITH_KNOTS ( 'NONE', 5,
 ( #27709, #27557, #13232, #20325, #1455, #8193, #23166, #13714, #11048, #22847, #30234, #8668, #18264, #25524, #1606 ),
 .UNSPECIFIED., .F., .F.,
 ( 6, 3, 3, 3, 6 ),
 ( 0.000000000000000000, 0.1000000000028630903, 0.3999999999999999667, 0.7000000000005727196, 1.000000000000000000 ),
 .UNSPECIFIED. ) ;
#21561=DIRECTION ( 'NONE',  ( 0.000000000000000000, -1.000000000000000000, 0.000000000000000000 ) ) ;
#21571=B_SPLINE_SURFACE_WITH_KNOTS ( 'NONE', 5, 1, ( 
 ( #14144, #6431 ),
 ( #25949, #11472 ),
 ( #30358, #18697 ),
 ( #6740, #2034 ),
 ( #11622, #26104 ),
 ( #23749, #26254 ),
 ( #2187, #21383 ),
 ( #30975, #9407 ),
 ( #19011, #4693 ),
 ( #14301, #18390 ),
 ( #16029, #25646 ),
 ( #4076, #10040 ),
 ( #3098, #12083 ),
 ( #27024, #24200 ),
 ( #457, #2495 ),
 ( #19793, #19328 ),
 ( #4855, #7818 ),
 ( #5003, #22150 ),
 ( #15068, #16957 ),
 ( #21691, #26562 ),
 ( #19335, #29376 ),
 ( #19482, #606 ),
 ( #19633, #21536 ),
 ( #9572, #302 ),
 ( #9881, #12392 ),
 ( #5147, #29219 ),
 ( #10193, #140 ),
 ( #24663, #2949 ),
 ( #2642, #28921 ),
 ( #17415, #9721 ) ),
 .UNSPECIFIED., .F., .F., .F.,
 ( 6, 3, 3, 3, 3, 3, 3, 3, 3, 6 ),
 ( 2, 2 ),
 ( 295.9469361829999912, 296.7817637200000149, 302.0406471359999614, 307.2995305649999978, 312.5584139889999733, 317.8172974060000229, 323.0761808360000487, 328.3350642730000004, 333.5939477180000381, 336.3523335059999795 ),
 ( -9.355471259890000464E-07, 0.7003637394550000783 ),
 .UNSPECIFIED. ) ;
#21584=CARTESIAN_POINT ( 'NONE',  ( -19.06889133170000150, 19.69230209619999883, 229.7995039799999972 ) ) ;
#21603=CARTESIAN_POINT ( 'NONE',  ( 22.41293933140000050, 16.47772227400000489, 222.9999999789999947 ) ) ;
#21610=CARTESIAN_POINT ( 'NONE',  ( 23.69119887980000172, 20.94188554260000146, 229.0000000000000000 ) ) ;
#21627=CARTESIAN_POINT ( 'NONE',  ( 26.80000000000000071, -6.394884621839999216E-14, 230.6999999999999886 ) ) ;
#21637=DIRECTION ( 'NONE',  ( 0.000000000000000000, 0.000000000000000000, 1.000000000000000000 ) ) ;
#21643=CARTESIAN_POINT ( 'NONE',  ( 26.49973092449999967, 5.074550867610000182, 230.6999999999999886 ) ) ;
#21655=CARTESIAN_POINT ( 'NONE',  ( 24.34123158960000310, -14.82477075300000102, 224.0987030360000176 ) ) ;
#21662=CARTESIAN_POINT ( 'NONE',  ( -8.249724945169999657, 8.807467740899999953, 231.9999989789999972 ) ) ;
#21663=CARTESIAN_POINT ( 'NONE',  ( -27.79999999990000248, 4.328052761030000362, 223.3999999999999773 ) ) ;
#21670=CARTESIAN_POINT ( 'NONE',  ( -4.960227444680000097, -16.90556345619999945, 230.0904314459999966 ) ) ;
#21679=CARTESIAN_POINT ( 'NONE',  ( 24.91921101730000032, -13.83103916669999833, 226.0027513979999867 ) ) ;
#21691=CARTESIAN_POINT ( 'NONE',  ( 11.88666889350000133, 2.326897762900000277, 231.9999991140000191 ) ) ;
#21713=ORIENTED_EDGE ( 'NONE', *, *, #19604, .T. ) ;
#21720=CARTESIAN_POINT ( 'NONE',  ( -0.03526712872449999647, -28.50022367440000082, 223.9000014189999774 ) ) ;
#21723=EDGE_CURVE ( 'NONE', #10448, #21281, #20315, .T. ) ;
#21740=EDGE_CURVE ( 'NONE', #28642, #29484, #21834, .T. ) ;
#21750=CARTESIAN_POINT ( 'NONE',  ( 25.20859211119999799, -13.29584934979999922, 225.3105417090000060 ) ) ;
#21756=VERTEX_POINT ( 'NONE', #12176 ) ;
#21761=CARTESIAN_POINT ( 'NONE',  ( -5.361385120500000490, 31.61859227569999931, 229.0000000000000000 ) ) ;
#21781=EDGE_CURVE ( 'NONE', #28642, #19036, #8659, .T. ) ;
#21782=CARTESIAN_POINT ( 'NONE',  ( 24.58947386300000204, 13.65571127169999954, 229.7313205199999686 ) ) ;
#21783=CARTESIAN_POINT ( 'NONE',  ( -7.957586915840000330, 16.45834648369999798, 230.6999999999999886 ) ) ;
#21784=ORIENTED_EDGE ( 'NONE', *, *, #10020, .T. ) ;
#21790=CONICAL_SURFACE ( 'NONE', #28315, 12.22526471199999598, 1.243158134259999770 ) ;
#21814=CARTESIAN_POINT ( 'NONE',  ( -9.117807398470000990, -8.314605678609998662, 232.6627643349999914 ) ) ;
#21815=CARTESIAN_POINT ( 'NONE',  ( -26.95773186790000153, 8.656139628340000058, 227.5999999999999943 ) ) ;
#21820=CARTESIAN_POINT ( 'NONE',  ( 24.60666973299075977, -12.93650480179744200, 224.8530246344855357 ) ) ;
#21825=CARTESIAN_POINT ( 'NONE',  ( 10.33059233208003214, -6.304462385806647973, 232.0000002394077399 ) ) ;
#21832=CARTESIAN_POINT ( 'NONE',  ( 24.55535052759999814, -13.03386662210000146, 225.5069763079999916 ) ) ;
#21834=B_SPLINE_CURVE_WITH_KNOTS ( 'NONE', 1,
 ( #23845, #18952 ),
 .UNSPECIFIED., .F., .F.,
 ( 2, 2 ),
 ( -3.500000000000000000, 3.500000000000000000 ),
 .UNSPECIFIED. ) ;
#21855=CARTESIAN_POINT ( 'NONE',  ( 27.29823224880000154, -6.039613253960000872E-14, 230.6577119970000069 ) ) ;
#21860=CARTESIAN_POINT ( 'NONE',  ( -0.9498500758684573775, -27.78406401609443321, 225.5583478121612870 ) ) ;
#21864=CARTESIAN_POINT ( 'NONE',  ( -24.60699806910000120, -12.93667933180000063, 224.8957833819999621 ) ) ;
#21871=CARTESIAN_POINT ( 'NONE',  ( -24.06944413539999772, 13.35197612260000000, 230.0000000000000000 ) ) ;
#21896=CARTESIAN_POINT ( 'NONE',  ( -23.58694728389455264, -14.71452256581467388, 224.4414045756103633 ) ) ;
#21932=EDGE_LOOP ( 'NONE', ( #26481, #12420, #22297, #21023, #28325 ) ) ;
#21951=B_SPLINE_SURFACE_WITH_KNOTS ( 'NONE', 5, 1, ( 
 ( #19288, #10427 ),
 ( #2458, #10578 ),
 ( #20173, #7891 ),
 ( #17642, #20019 ),
 ( #17498, #28881 ),
 ( #26523, #7172 ),
 ( #26217, #4654 ),
 ( #21655, #16915 ),
 ( #9535, #7330 ),
 ( #24744, #27255 ),
 ( #104, #12934 ),
 ( #24904, #16760 ),
 ( #21494, #19877 ),
 ( #11891, #14262 ),
 ( #12050, #4963 ) ),
 .UNSPECIFIED., .F., .F., .F.,
 ( 6, 3, 3, 3, 6 ),
 ( 2, 2 ),
 ( 0.000000000000000000, 0.5238999881929999880, 1.047799976380000109, 1.571699964580000053, 1.746333293980000034 ),
 ( -0.7000000000009999335, 2.555864960449999711E-06 ),
 .UNSPECIFIED. ) ;
#21972=CARTESIAN_POINT ( 'NONE',  ( -8.404590197819999275, 8.972803037040000262, 232.6627643349999914 ) ) ;
#21974=CARTESIAN_POINT ( 'NONE',  ( -11.07235429843649754, 4.885731407866478193, 232.0000000000049170 ) ) ;
#21997=EDGE_LOOP ( 'NONE', ( #21190, #22992, #15850, #12922 ) ) ;
#22005=CARTESIAN_POINT ( 'NONE',  ( 27.04041630560000087, -7.083781863679999624, 230.6999999999999886 ) ) ;
#22017=B_SPLINE_SURFACE_WITH_KNOTS ( 'NONE', 5, 1, ( 
 ( #6833, #26042 ),
 ( #19686, #12293 ),
 ( #1817, #12437 ),
 ( #17318, #22057 ),
 ( #508, #29271 ),
 ( #25892, #4327 ),
 ( #23533, #11563 ),
 ( #18786, #29585 ),
 ( #1266, #25020 ),
 ( #3002, #27525 ),
 ( #22362, #5820 ),
 ( #12594, #12907 ),
 ( #25175, #12747 ),
 ( #20450, #30046 ),
 ( #8321, #24713 ) ),
 .UNSPECIFIED., .F., .F., .F.,
 ( 6, 3, 3, 3, 6 ),
 ( 2, 2 ),
 ( 0.000000000000000000, 0.5239017171269999551, 1.047803434249999999, 1.571705151379999998, 1.746339057089999924 ),
 ( -0.7000000000009999335, 2.556331299420000144E-06 ),
 .UNSPECIFIED. ) ;
#22024=CARTESIAN_POINT ( 'NONE',  ( -21.44011192940000399, 17.18091426960000234, 229.9751246980000019 ) ) ;
#22028=EDGE_LOOP ( 'NONE', ( #16752, #11559, #1145, #9648 ) ) ;
#22037=CARTESIAN_POINT ( 'NONE',  ( 19.20676039538625446, 20.00032347732748761, 230.4273714388203587 ) ) ;
#22048=CARTESIAN_POINT ( 'NONE',  ( -23.50695067597005661, -14.84192170558070956, 224.8529579040860256 ) ) ;
#22057=CARTESIAN_POINT ( 'NONE',  ( 1.063086518149999993, -27.77985718819999761, 225.3101849020000031 ) ) ;
#22059=CARTESIAN_POINT ( 'NONE',  ( 24.68173674080000168, -14.25001227039999918, 223.9000014189999774 ) ) ;
#22075=DIRECTION ( 'NONE',  ( 0.000000000000000000, 0.000000000000000000, 1.000000000000000000 ) ) ;
#22083=EDGE_CURVE ( 'NONE', #2003, #7240, #28177, .T. ) ;
#22094=CARTESIAN_POINT ( 'NONE',  ( 27.71720220719999972, 4.680497606070000316, 229.4485730569999760 ) ) ;
#22102=ORIENTED_EDGE ( 'NONE', *, *, #3864, .T. ) ;
#22121=CARTESIAN_POINT ( 'NONE',  ( -8.949800212739999594, -8.161398505059999309, 231.9999989789999972 ) ) ;
#22135=ORIENTED_EDGE ( 'NONE', *, *, #27513, .T. ) ;
#22138=CARTESIAN_POINT ( 'NONE',  ( 24.87112161019999945, -13.91739822849999975, 226.0424756639999941 ) ) ;
#22143=CARTESIAN_POINT ( 'NONE',  ( -25.90993013099999942, 13.08108041899999918, 229.0000000000000000 ) ) ;
#22150=CARTESIAN_POINT ( 'NONE',  ( 12.26718592479999970, -0.8151587190580000808, 232.6627648150000027 ) ) ;
#22157=ADVANCED_FACE ( 'NONE', ( #14050 ), #24265, .T. ) ;
#22168=CARTESIAN_POINT ( 'NONE',  ( -18.50402760634471377, 20.00005619007534463, 230.6403179726253541 ) ) ;
#22169=CARTESIAN_POINT ( 'NONE',  ( -21.93401131390000103, 17.57670095970000190, 229.4485730019999892 ) ) ;
#22180=ORIENTED_EDGE ( 'NONE', *, *, #21187, .F. ) ;
#22182=ORIENTED_EDGE ( 'NONE', *, *, #24808, .T. ) ;
#22187=EDGE_CURVE ( 'NONE', #24425, #26590, #11791, .T. ) ;
#22206=CARTESIAN_POINT ( 'NONE',  ( 3.550686847520000117E-05, -28.50022181210000127, 223.9000014189999774 ) ) ;
#22219=ORIENTED_EDGE ( 'NONE', *, *, #2903, .F. ) ;
#22221=CARTESIAN_POINT ( 'NONE',  ( 25.04666666270000164, 13.90965967079999999, 230.2432540810000319 ) ) ;
#22223=AXIS2_PLACEMENT_3D ( 'NONE', #20288, #15415, #25330 ) ;
#22235=CARTESIAN_POINT ( 'NONE',  ( 5.229687933670000177, -30.84198039099999633, 228.9999999970000317 ) ) ;
#22242=CARTESIAN_POINT ( 'NONE',  ( 17.83931934289999788, 20.00000000000000000, 230.0000000000000000 ) ) ;
#22272=CARTESIAN_POINT ( 'NONE',  ( -11.76358722600000029, -3.726270779419999624, 232.6627643349999914 ) ) ;
#22274=B_SPLINE_CURVE_WITH_KNOTS ( 'NONE', 5,
 ( #10317, #1337, #17536, #17990, #20524, #30125, #8554, #3217, #6203, #29498, #12827, #7935, #22429, #27145, #5580 ),
 .UNSPECIFIED., .F., .F.,
 ( 6, 3, 3, 3, 6 ),
 ( 0.000000000000000000, 0.2000000000000000111, 0.3999999999986155186, 0.6999999999975770049, 1.000000000000000000 ),
 .UNSPECIFIED. ) ;
#22275=CARTESIAN_POINT ( 'NONE',  ( -10.33059293845328241, 6.304462755849592703, 232.0000000000049738 ) ) ;
#22291=CARTESIAN_POINT ( 'NONE',  ( -24.60699806910000120, -12.93667933180000063, 225.0000014190000002 ) ) ;
#22295=ORIENTED_EDGE ( 'NONE', *, *, #25276, .T. ) ;
#22297=ORIENTED_EDGE ( 'NONE', *, *, #6762, .T. ) ;
#22321=CARTESIAN_POINT ( 'NONE',  ( -18.23049700918086202, 20.00000270586327389, 230.6797159284481324 ) ) ;
#22323=CARTESIAN_POINT ( 'NONE',  ( -26.80000000000000071, -7.460698725479998033E-14, 230.0000000000000000 ) ) ;
#22340=CARTESIAN_POINT ( 'NONE',  ( 23.95489023949999918, -14.10735628980000023, 226.0798541909999813 ) ) ;
#22356=DIRECTION ( 'NONE',  ( 0.000000000000000000, 0.000000000000000000, 1.000000000000000000 ) ) ;
#22362=CARTESIAN_POINT ( 'NONE',  ( 0.2462945485050000161, -28.49939181889999773, 226.0797949779999954 ) ) ;
#22366=CARTESIAN_POINT ( 'NONE',  ( 1.127732790480000080, -28.47784299079999926, 224.8959500220000223 ) ) ;
#22368=CIRCLE ( 'NONE', #20867, 0.9999999999999982236 ) ;
#22386=CARTESIAN_POINT ( 'NONE',  ( -3.378474373710000034, -11.51459555979999827, 232.0000000000000000 ) ) ;
#22387=CARTESIAN_POINT ( 'NONE',  ( -19.80526803560000104, 19.50877411510000314, 228.1999999999999886 ) ) ;
#22422=CARTESIAN_POINT ( 'NONE',  ( -13.73802074570000009, -27.58422840009999888, 229.2930759660000035 ) ) ;
#22426=CARTESIAN_POINT ( 'NONE',  ( -20.30396346370000060, 20.00000000000000000, 227.0000000000000000 ) ) ;
#22429=CARTESIAN_POINT ( 'NONE',  ( 18.15340080560000047, 19.92139761430000178, 229.9929672670000116 ) ) ;
#22443=CARTESIAN_POINT ( 'NONE',  ( 23.69119887980000172, 20.94188554260000146, 229.0000000000000000 ) ) ;
#22446=DIRECTION ( 'NONE',  ( 1.000000000000000000, 0.000000000000000000, 0.000000000000000000 ) ) ;
#22478=CARTESIAN_POINT ( 'NONE',  ( -19.98328564520809891, 20.00005048715008726, 229.8503962144677359 ) ) ;
#22501=CARTESIAN_POINT ( 'NONE',  ( -23.55406855550000245, 16.04544956020000157, 222.0000000000000000 ) ) ;
#22515=CARTESIAN_POINT ( 'NONE',  ( -28.35924375250000296, -1.754620794519999711E-14, 229.7625741969999922 ) ) ;
#22532=ORIENTED_EDGE ( 'NONE', *, *, #19923, .T. ) ;
#22536=LINE ( 'NONE', #827, #6423 ) ;
#22537=CARTESIAN_POINT ( 'NONE',  ( -26.05511412830000140, 14.93229958979999950, 222.0000000000000000 ) ) ;
#22540=CARTESIAN_POINT ( 'NONE',  ( -20.30396346370000060, 20.00000000000000000, 227.8000000000000114 ) ) ;
#22557=CARTESIAN_POINT ( 'NONE',  ( 16.30906683129999735, -8.426343777580001415, 230.6999999999999886 ) ) ;
#22575=CARTESIAN_POINT ( 'NONE',  ( -27.77512470430000135, 2.245670316370000201E-11, 229.2930777930000090 ) ) ;
#22578=EDGE_CURVE ( 'NONE', #10061, #14789, #742, .T. ) ;
#22586=CARTESIAN_POINT ( 'NONE',  ( 7.908785388650001025, 16.35326433119999834, 231.6999999999999886 ) ) ;
#22592=FACE_OUTER_BOUND ( 'NONE', #7550, .T. ) ;
#22601=CARTESIAN_POINT ( 'NONE',  ( 28.50000000000000000, 8.881784197000000993E-16, 222.0000000000000000 ) ) ;
#22610=CARTESIAN_POINT ( 'NONE',  ( 18.34331631877363122, 20.00003010481418286, 230.6660856982278176 ) ) ;
#22659=CARTESIAN_POINT ( 'NONE',  ( -24.07583586439999834, -13.90018868249999962, 226.1000014189999945 ) ) ;
#22672=CARTESIAN_POINT ( 'NONE',  ( -25.20890834729999952, -13.29605215849999844, 224.6893543200000067 ) ) ;
#22680=CARTESIAN_POINT ( 'NONE',  ( 26.07656786439999763, 9.132422599079999870, 230.6999999999999886 ) ) ;
#22684=CARTESIAN_POINT ( 'NONE',  ( -19.80526803560000104, 19.50877411510000314, 227.3999999999999773 ) ) ;
#22689=EDGE_LOOP ( 'NONE', ( #7463, #26401, #3477, #29161 ) ) ;
#22694=CARTESIAN_POINT ( 'NONE',  ( -1.127665019380000189, -28.47796022459999676, 225.0000014190000002 ) ) ;
#22697=CARTESIAN_POINT ( 'NONE',  ( -28.45771199710000232, 4.798408318400000816, 229.4982322489999831 ) ) ;
#22701=CARTESIAN_POINT ( 'NONE',  ( -26.49971571929999925, -5.074679369350000080, 230.6999999999999886 ) ) ;
#22706=B_SPLINE_CURVE_WITH_KNOTS ( 'NONE', 5,
 ( #6315, #28020, #16220, #6464, #28178, #30701 ),
 .UNSPECIFIED., .F., .F.,
 ( 6, 6 ),
 ( 66.69070842060000359, 88.33140247330000250 ),
 .UNSPECIFIED. ) ;
#22721=EDGE_CURVE ( 'NONE', #13075, #6979, #23680, .T. ) ;
#22730=ADVANCED_FACE ( 'NONE', ( #3829 ), #18345, .F. ) ;
#22734=CARTESIAN_POINT ( 'NONE',  ( 25.00924755590000004, -13.66774366000000107, 224.0987054560000047 ) ) ;
#22736=CARTESIAN_POINT ( 'NONE',  ( 5.361384718770000113, -31.61859215249999977, 222.0000000000000000 ) ) ;
#22738=B_SPLINE_CURVE_WITH_KNOTS ( 'NONE', 5,
 ( #25618, #6252, #1381, #13804, #20730, #30329, #13484, #13329, #22772, #15855, #11291, #27803, #8760, #20412, #13647 ),
 .UNSPECIFIED., .F., .F.,
 ( 6, 3, 3, 3, 6 ),
 ( 0.000000000000000000, 0.2999999999999999889, 0.6000000000034357850, 0.8999999999994273692, 1.000000000000000000 ),
 .UNSPECIFIED. ) ;
#22745=CARTESIAN_POINT ( 'NONE',  ( 27.79999999999999716, -2.355449169040000061E-11, 229.0000000000000000 ) ) ;
#22747=EDGE_CURVE ( 'NONE', #7240, #4391, #804, .T. ) ;
#22765=LINE ( 'NONE', #27178, #18543 ) ;
#22772=CARTESIAN_POINT ( 'NONE',  ( -24.43799431770000297, -14.66523353640000060, 226.0028091380000035 ) ) ;
#22777=CARTESIAN_POINT ( 'NONE',  ( -23.58385914817347384, -14.71952726119423716, 225.5626237715469529 ) ) ;
#22781=CARTESIAN_POINT ( 'NONE',  ( -20.09104791241940546, 19.99996880304969693, 229.7041693757062717 ) ) ;
#22833=SHAPE_REPRESENTATION ( 'Front End Cap', ( #17722 ), #25295 ) ;
#22835=CARTESIAN_POINT ( 'NONE',  ( 17.99935157089999649, 20.17941515460000090, 230.6999999999999886 ) ) ;
#22847=CARTESIAN_POINT ( 'NONE',  ( -0.8958568848300000331, -28.48628573779999940, 225.6801695290000112 ) ) ;
#22853=AXIS2_PLACEMENT_3D ( 'NONE', #30910, #21465, #17043 ) ;
#22857=CARTESIAN_POINT ( 'NONE',  ( -28.04325408110000240, 8.622238390189998484E-15, 230.2432540810000319 ) ) ;
#22858=CARTESIAN_POINT ( 'NONE',  ( -27.79999999999999716, -2.354540544949999935E-11, 222.0000000000000000 ) ) ;
#22862=CARTESIAN_POINT ( 'NONE',  ( -27.79999999999999716, 2.356514983149999809E-11, 222.0000000000000000 ) ) ;
#22863=CARTESIAN_POINT ( 'NONE',  ( 2.797823115279999939, -26.80098304230000039, 230.6999999999999886 ) ) ;
#22868=CARTESIAN_POINT ( 'NONE',  ( 20.30405755279999980, 20.00000000000000000, 229.0000000000000000 ) ) ;
#22876=EDGE_CURVE ( 'NONE', #18537, #10995, #13553, .T. ) ;
#22885=CARTESIAN_POINT ( 'NONE',  ( -23.04052943119999952, -20.36665827710000087, 229.4485687169999721 ) ) ;
#22894=PRODUCT_DEFINITION_SHAPE ( 'NONE', 'NONE',  #8875 ) ;
#22897=CARTESIAN_POINT ( 'NONE',  ( 24.26025373720000289, -13.57556515269999942, 223.9575271749999672 ) ) ;
#22908=ORIENTED_EDGE ( 'NONE', *, *, #22876, .F. ) ;
#22910=CARTESIAN_POINT ( 'NONE',  ( 27.79999999999999716, -2.355691128989999990E-11, 226.2000000000000171 ) ) ;
#22930=EDGE_CURVE ( 'NONE', #18537, #29947, #24778, .T. ) ;
#22945=CARTESIAN_POINT ( 'NONE',  ( -20.30396346370000060, 20.00000000000000000, 229.0000000000000000 ) ) ;
#22946=CARTESIAN_POINT ( 'NONE',  ( -20.28212397553859603, 20.00001296311320687, 229.2653906922940621 ) ) ;
#22956=EDGE_LOOP ( 'NONE', ( #19227, #13503, #2558, #30826 ) ) ;
#22959=CARTESIAN_POINT ( 'NONE',  ( 23.50667118420000179, -14.84174322970000048, 225.0000014190000002 ) ) ;
#22963=CARTESIAN_POINT ( 'NONE',  ( 2.131628207279999844E-14, -1.704192342799999938E-14, 231.6999999999999886 ) ) ;
#22969=EDGE_CURVE ( 'NONE', #17736, #19467, #27757, .T. ) ;
#22988=CARTESIAN_POINT ( 'NONE',  ( -24.58975347950000057, -12.96948186770000078, 224.6893543200000067 ) ) ;
#22992=ORIENTED_EDGE ( 'NONE', *, *, #12412, .F. ) ;
#22998=CARTESIAN_POINT ( 'NONE',  ( -24.07583586439999834, -13.90018868249999962, 226.1000014189999945 ) ) ;
#23003=ORIENTED_EDGE ( 'NONE', *, *, #16155, .T. ) ;
#23017=CARTESIAN_POINT ( 'NONE',  ( -27.48714010850000022, 9.611077580710000845, 229.2404163060000144 ) ) ;
#23021=FACE_BOUND ( 'NONE', #9482, .T. ) ;
#23022=CARTESIAN_POINT ( 'NONE',  ( 26.63560679380000096, -3.754777938270000170, 230.6999999999999886 ) ) ;
#23026=CARTESIAN_POINT ( 'NONE',  ( 20.30405755279999980, 20.00000000000000000, 228.1999999569999886 ) ) ;
#23046=CARTESIAN_POINT ( 'NONE',  ( -22.65095495759999977, -20.02231963160000205, 229.9172003479999660 ) ) ;
#23057=CARTESIAN_POINT ( 'NONE',  ( 24.07552037900000030, -13.90000980950000020, 223.9000014189999774 ) ) ;
#23060=CARTESIAN_POINT ( 'NONE',  ( -28.46654375369999812, 1.746771098880000261, 222.0000000000000000 ) ) ;
#23070=CARTESIAN_POINT ( 'NONE',  ( 22.83442928010000017, 16.43389279790000046, 227.5999999999999943 ) ) ;
#23081=CARTESIAN_POINT ( 'NONE',  ( 20.21755947467096348, 19.99998237122240496, 229.4578303307542910 ) ) ;
#23093=CARTESIAN_POINT ( 'NONE',  ( -24.68204616399999907, -14.25020164319999871, 226.1000014189999945 ) ) ;
#23128=CARTESIAN_POINT ( 'NONE',  ( -27.79999999970000246, -10.21376199200000201, 222.0000000000000000 ) ) ;
#23149=EDGE_CURVE ( 'NONE', #17135, #29716, #23659, .T. ) ;
#23150=CARTESIAN_POINT ( 'NONE',  ( -28.50000000000000000, 1.776356839399999922E-14, 222.0000000000000000 ) ) ;
#23157=CARTESIAN_POINT ( 'NONE',  ( 18.66688684140000376, 20.92780155799999875, 230.2432540810000319 ) ) ;
#23166=CARTESIAN_POINT ( 'NONE',  ( -0.4820778520819999913, -28.49640832880000119, 226.0025182780000250 ) ) ;
#23182=ORIENTED_EDGE ( 'NONE', *, *, #21008, .T. ) ;
#23199=CARTESIAN_POINT ( 'NONE',  ( 20.58567524440000085, -20.71744736909999673, 229.4485717599999930 ) ) ;
#23203=CARTESIAN_POINT ( 'NONE',  ( 10.70777106509999932, -25.82052991099999772, 222.0000000000000000 ) ) ;
#23204=CARTESIAN_POINT ( 'NONE',  ( -5.114260856059999583, -17.43050419540000107, 230.6999999999999886 ) ) ;
#23213=CARTESIAN_POINT ( 'NONE',  ( 28.49999999970000175, -7.466149220240000162, 229.0000000000000000 ) ) ;
#23215=CARTESIAN_POINT ( 'NONE',  ( 17.83931934289999788, 20.00000000000000000, 230.6999999999999886 ) ) ;
#23221=CARTESIAN_POINT ( 'NONE',  ( 25.26809617030000155, 12.77001320659999983, 229.0000000000000000 ) ) ;
#23227=FILL_AREA_STYLE ('',( #16133 ) ) ;
#23232=CARTESIAN_POINT ( 'NONE',  ( 17.83931934289999788, 20.00000000000000000, 230.6999999999999886 ) ) ;
#23242=FACE_BOUND ( 'NONE', #4105, .T. ) ;
#23248=CARTESIAN_POINT ( 'NONE',  ( -3.868754989949999779, 11.66966430080000094, 232.6627643349999914 ) ) ;
#23252=CARTESIAN_POINT ( 'NONE',  ( -1.100001419170000050, -27.77850706310000106, 225.1040592169999854 ) ) ;
#23281=CARTESIAN_POINT ( 'NONE',  ( -26.80000000000000071, 3.552713678799999608E-15, 230.6999999999999886 ) ) ;
#23288=CARTESIAN_POINT ( 'NONE',  ( 1.127732790480000080, -28.47784299079999926, 224.8959500220000223 ) ) ;
#23308=CARTESIAN_POINT ( 'NONE',  ( 22.43614352489999675, 17.98932536259999893, 229.7625741969999922 ) ) ;
#23311=CARTESIAN_POINT ( 'NONE',  ( -24.11017618899999704, -13.84060607850000046, 226.0986578700000109 ) ) ;
#23333=CARTESIAN_POINT ( 'NONE',  ( -24.48873108229999929, -14.58042505439999914, 226.0425106499999970 ) ) ;
#23347=CARTESIAN_POINT ( 'NONE',  ( -25.22658730140000216, -13.26242337740000110, 225.1042194559999814 ) ) ;
#23355=DIRECTION ( 'NONE',  ( -0.9595496299847263710, 0.2815395311429191305, 0.000000000000000000 ) ) ;
#23362=CARTESIAN_POINT ( 'NONE',  ( 5.041582825300000792, -29.73257086209999756, 230.0000000000000000 ) ) ;
#23365=CARTESIAN_POINT ( 'NONE',  ( -3.339220672710000226, -27.75291293060000086, 222.0000000000000000 ) ) ;
#23375=CARTESIAN_POINT ( 'NONE',  ( 4.977446931567997446, 11.28020582389469517, 232.6627635322004153 ) ) ;
#23376=VERTEX_POINT ( 'NONE', #25821 ) ;
#23390=CARTESIAN_POINT ( 'NONE',  ( 22.83442928019999840, 16.43389279790000046, 222.0000000000000000 ) ) ;
#23396=PRESENTATION_STYLE_ASSIGNMENT (( #9051 ) ) ;
#23409=FACE_OUTER_BOUND ( 'NONE', #22028, .T. ) ;
#23416=CARTESIAN_POINT ( 'NONE',  ( 20.30406631259999983, 20.00000862929999812, 229.0000000000000000 ) ) ;
#23426=CARTESIAN_POINT ( 'NONE',  ( 20.30405755279999980, 20.00000000000000000, 226.9999998930000231 ) ) ;
#23437=ORIENTED_EDGE ( 'NONE', *, *, #18840, .T. ) ;
#23448=CARTESIAN_POINT ( 'NONE',  ( -27.04041630560000087, -3.552713678799999608E-15, 230.6999999999999886 ) ) ;
#23454=CARTESIAN_POINT ( 'NONE',  ( 0.8738980057240000043, -27.78653623639999992, 224.3198498209999912 ) ) ;
#23471=CARTESIAN_POINT ( 'NONE',  ( 21.80586599240000112, 17.48396816709999868, 230.5592437530000041 ) ) ;
#23476=EDGE_CURVE ( 'NONE', #13298, #11678, #11813, .T. ) ;
#23483=ORIENTED_EDGE ( 'NONE', *, *, #23149, .T. ) ;
#23492=CARTESIAN_POINT ( 'NONE',  ( -24.07583586439999834, -13.90018868249999962, 226.1000014189999945 ) ) ;
#23496=CARTESIAN_POINT ( 'NONE',  ( 27.79999999999999716, 2.355804440410000085E-11, 229.0000000000000000 ) ) ;
#23511=B_SPLINE_SURFACE_WITH_KNOTS ( 'NONE', 5, 1, ( 
 ( #13432, #30275 ),
 ( #10462, #5729 ),
 ( #1022, #10610 ),
 ( #29796, #8228 ),
 ( #4469, #11394 ),
 ( #16261, #30743 ),
 ( #16110, #28535 ),
 ( #14068, #1644 ),
 ( #15956, #8863 ),
 ( #9492, #30597 ),
 ( #18468, #9333 ),
 ( #6822, #23365 ),
 ( #16420, #11234 ),
 ( #21147, #23827 ),
 ( #26029, #28066 ),
 ( #4613, #23203 ),
 ( #14221, #6982 ),
 ( #30443, #23673 ),
 ( #6662, #2107 ),
 ( #11700, #18933 ),
 ( #4315, #4156 ),
 ( #16571, #6510 ),
 ( #30904, #21303 ),
 ( #28220, #26177 ),
 ( #31056, #19094 ),
 ( #9173, #2271 ),
 ( #13911, #11857 ) ),
 .UNSPECIFIED., .F., .F., .F.,
 ( 6, 3, 3, 3, 3, 3, 3, 3, 6 ),
 ( 2, 2 ),
 ( 0.000000000000000000, 12.04914910469999967, 24.12830621100000172, 36.22018076730000047, 48.28758829720000278, 60.33208762030000116, 72.38455155859999479, 84.43687076610000020, 88.75867308210000317 ),
 ( -2.393070191420000080E-05, 0.7036780443879999680 ),
 .UNSPECIFIED. ) ;
#23533=CARTESIAN_POINT ( 'NONE',  ( 0.8260714174469999671, -28.48835664879999996, 225.7596297540000023 ) ) ;
#23550=CARTESIAN_POINT ( 'NONE',  ( -12.32633706535996154, 0.2818134420149785435, 232.6627637660202197 ) ) ;
#23557=ADVANCED_FACE ( 'NONE', ( #28587 ), #16970, .T. ) ;
#23572=CARTESIAN_POINT ( 'NONE',  ( 19.79266700209999996, 19.51190850369999907, 229.1494847489999813 ) ) ;
#23573=CARTESIAN_POINT ( 'NONE',  ( -19.80526803549999926, 19.50877411510000314, 229.0000000000000000 ) ) ;
#23574=B_SPLINE_CURVE_WITH_KNOTS ( 'NONE', 3,
 ( #30161, #10240, #8433, #27801, #10973, #29424, #17462, #15681, #10393, #2839, #12434, #25456 ),
 .UNSPECIFIED., .F., .F.,
 ( 4, 2, 2, 2, 2, 4 ),
 ( 0.000000000000000000, 0.1249999999999999445, 0.2499999999999998890, 0.5000000000000000000, 0.7500000000000001110, 1.000000000000000000 ),
 .UNSPECIFIED. ) ;
#23576=CARTESIAN_POINT ( 'NONE',  ( -0.3738033647169999862, -27.79799560440000050, 226.0423263479999889 ) ) ;
#23599=CARTESIAN_POINT ( 'NONE',  ( -24.68204616399999907, -14.25020164319999871, 223.9000014189999774 ) ) ;
#23602=CARTESIAN_POINT ( 'NONE',  ( -13.50216071430000042, -27.11059322570000418, 230.6577119970000069 ) ) ;
#23606=CARTESIAN_POINT ( 'NONE',  ( -1.100001242879427243, -27.77850260588756015, 225.1469357386177421 ) ) ;
#23622=ORIENTED_EDGE ( 'NONE', *, *, #19968, .F. ) ;
#23631=CARTESIAN_POINT ( 'NONE',  ( -24.60699806910000120, -12.93667933180000063, 225.1042194559999814 ) ) ;
#23645=CARTESIAN_POINT ( 'NONE',  ( -24.15901410609999900, -15.12012600319999933, 225.5071239680000303 ) ) ;
#23659=B_SPLINE_CURVE_WITH_KNOTS ( 'NONE', 1,
 ( #29748, #14830 ),
 .UNSPECIFIED., .F., .F.,
 ( 2, 2 ),
 ( -0.7031447686210000603, -5.021915139291621699E-08 ),
 .UNSPECIFIED. ) ;
#23662=ORIENTED_EDGE ( 'NONE', *, *, #28939, .T. ) ;
#23664=EDGE_LOOP ( 'NONE', ( #15039, #484, #13388, #15095 ) ) ;
#23670=CARTESIAN_POINT ( 'NONE',  ( 25.33947091559999976, -14.52216050880000076, 229.4485726019999845 ) ) ;
#23673=CARTESIAN_POINT ( 'NONE',  ( 18.73270429609999965, -20.74707689250000087, 222.0000000000000000 ) ) ;
#23675=ORIENTED_EDGE ( 'NONE', *, *, #3105, .T. ) ;
#23680=B_SPLINE_CURVE_WITH_KNOTS ( 'NONE', 5,
 ( #16095, #18131, #18453, #8847, #18291, #1630, #28051, #11220, #20346, #3658, #27898, #27733, #15779, #23347, #1790 ),
 .UNSPECIFIED., .F., .F.,
 ( 6, 3, 3, 3, 6 ),
 ( 0.000000000000000000, 0.1000000000022905483, 0.4000000000034356629, 0.7000000000005726086, 1.000000000000000000 ),
 .UNSPECIFIED. ) ;
#23688=EDGE_CURVE ( 'NONE', #17409, #18614, #27324, .T. ) ;
#23689=CARTESIAN_POINT ( 'NONE',  ( -24.68204616399999907, -14.25020164319999871, 223.9000014189999774 ) ) ;
#23717=CARTESIAN_POINT ( 'NONE',  ( 24.09856112909999837, -15.21545593799999985, 225.1041867410000350 ) ) ;
#23718=FACE_OUTER_BOUND ( 'NONE', #19257, .T. ) ;
#23719=CARTESIAN_POINT ( 'NONE',  ( -19.80526803560000104, 19.50877411520000138, 223.3999999999999773 ) ) ;
#23722=CARTESIAN_POINT ( 'NONE',  ( -0.06887222117140000266, -27.80017212539999960, 226.0986539140000104 ) ) ;
#23732=CARTESIAN_POINT ( 'NONE',  ( -27.79999999999999716, -2.358405305979999929E-11, 229.1414213560000235 ) ) ;
#23748=B_SPLINE_CURVE_WITH_KNOTS ( 'NONE', 5,
 ( #21272, #8833, #6795, #18906, #1775, #21433 ),
 .UNSPECIFIED., .F., .F.,
 ( 6, 6 ),
 ( -88.61406016669999985, -71.78006588680000277 ),
 .UNSPECIFIED. ) ;
#23749=CARTESIAN_POINT ( 'NONE',  ( -2.703235379809999728, -11.76103604130000058, 231.9999991140000191 ) ) ;
#23753=CARTESIAN_POINT ( 'NONE',  ( 20.82782576890000215, -20.96114668230000078, 230.2432540810000319 ) ) ;
#23757=CARTESIAN_POINT ( 'NONE',  ( 19.80538173169999894, 19.50875421069999760, 226.9999998930000231 ) ) ;
#23760=CARTESIAN_POINT ( 'NONE',  ( -24.55564696219999732, -13.03410599059999875, 224.4928762930000232 ) ) ;
#23763=CARTESIAN_POINT ( 'NONE',  ( 7.908785388650001025, 16.35326433119999834, 231.6999999999999886 ) ) ;
#23779=CARTESIAN_POINT ( 'NONE',  ( 3.550686847520000117E-05, -28.50022181210000127, 223.9000014189999774 ) ) ;
#23782=CARTESIAN_POINT ( 'NONE',  ( 23.50666810109999716, -14.84174128299999929, 225.1041867410000350 ) ) ;
#23788=CARTESIAN_POINT ( 'NONE',  ( -20.25360388639999698, 20.00000774629999611, 229.3817167830000017 ) ) ;
#23810=CARTESIAN_POINT ( 'NONE',  ( 25.22625794089999829, -13.26224522399999906, 225.1041818340000020 ) ) ;
#23817=CARTESIAN_POINT ( 'NONE',  ( 28.49999999959999641, 10.47094317839999889, 229.0000000000000000 ) ) ;
#23818=EDGE_CURVE ( 'NONE', #16560, #13298, #19067, .T. ) ;
#23826=CARTESIAN_POINT ( 'NONE',  ( 24.21598885539167867, -13.65447905993845978, 226.0728589708802474 ) ) ;
#23827=CARTESIAN_POINT ( 'NONE',  ( 3.820026707160000257, -27.79243965350000067, 222.0000000000000000 ) ) ;
#23828=CARTESIAN_POINT ( 'NONE',  ( 0.6686231747779999290, -28.49266848160000265, 225.9009072510000067 ) ) ;
#23845=CARTESIAN_POINT ( 'NONE',  ( 27.79999999999999716, 2.355804440410000085E-11, 229.0000000000000000 ) ) ;
#23853=CARTESIAN_POINT ( 'NONE',  ( 24.31679662959999888, 11.82640008669999965, 230.6999999999999886 ) ) ;
#23868=B_SPLINE_CURVE_WITH_KNOTS ( 'NONE', 3,
 ( #4361, #13964, #11598, #21196, #7791, #880, #24328, #22275, #21974, #14732, #29042, #10324, #14892, #17392, #15044, #429, #12514, #8092 ),
 .UNSPECIFIED., .F., .F.,
 ( 4, 2, 2, 2, 2, 2, 2, 2, 4 ),
 ( 0.000000000000000000, 0.1249999999999999722, 0.2499999999999999445, 0.3749999999999998890, 0.4999999999999998890, 0.6249999999999998890, 0.7499999999999997780, 0.8749999999999998890, 1.000000000000000000 ),
 .UNSPECIFIED. ) ;
#23876=CARTESIAN_POINT ( 'NONE',  ( 0.3105039177659999483, 12.06370740949999920, 231.9999989789999972 ) ) ;
#23877=CARTESIAN_POINT ( 'NONE',  ( -19.80526803549999926, 19.50877411510000314, 227.5999999999999943 ) ) ;
#23891=ORIENTED_EDGE ( 'NONE', *, *, #19416, .T. ) ;
#23892=VECTOR ( 'NONE', #22446, 1000.000000000000000 ) ;
#23898=VERTEX_POINT ( 'NONE', #8097 ) ;
#23900=B_SPLINE_CURVE_WITH_KNOTS ( 'NONE', 5,
 ( #11170, #11331, #13368, #3935, #18403, #6293 ),
 .UNSPECIFIED., .F., .F.,
 ( 6, 6 ),
 ( 76.73731126729998664, 94.75474465359999954 ),
 .UNSPECIFIED. ) ;
#23902=CARTESIAN_POINT ( 'NONE',  ( -28.50000000000000000, -5.684341886079999373E-14, 229.0000000000000000 ) ) ;
#23913=CARTESIAN_POINT ( 'NONE',  ( -28.45771199689999875, -10.45540640809999999, 229.4982322489999831 ) ) ;
#23915=CARTESIAN_POINT ( 'NONE',  ( -24.11911872370000154, -15.18353100999999938, 224.6893563800000209 ) ) ;
#23918=CARTESIAN_POINT ( 'NONE',  ( -27.79999999999999716, -2.355663498000000066E-11, 223.3999999999999773 ) ) ;
#23930=PLANE ( 'NONE',  #15197 ) ;
#23935=ORIENTED_EDGE ( 'NONE', *, *, #20743, .F. ) ;
#23941=CARTESIAN_POINT ( 'NONE',  ( 23.56533302370000271, -14.74861233630000079, 225.5069924249999929 ) ) ;
#23952=ORIENTED_EDGE ( 'NONE', *, *, #19604, .F. ) ;
#23967=CARTESIAN_POINT ( 'NONE',  ( 24.91921101730000032, -13.83103916669999833, 226.0027513979999867 ) ) ;
#23968=CARTESIAN_POINT ( 'NONE',  ( 20.30405756109999871, 20.00000000820000068, 226.9999998930000231 ) ) ;
#23970=ORIENTED_EDGE ( 'NONE', *, *, #8642, .F. ) ;
#23996=CARTESIAN_POINT ( 'NONE',  ( 27.77512470430000135, -2.242274238020000225E-11, 229.2930777930000090 ) ) ;
#23997=CARTESIAN_POINT ( 'NONE',  ( -17.50139837460000081, 5.282193806050000440, 230.6999999999999886 ) ) ;
#24024=CARTESIAN_POINT ( 'NONE',  ( -10.37415685080000038, -6.597363088169999834, 232.6627643349999914 ) ) ;
#24025=CARTESIAN_POINT ( 'NONE',  ( -27.79999999990000248, 4.328052761030000362, 227.5999999999999943 ) ) ;
#24028=CARTESIAN_POINT ( 'NONE',  ( 24.21557264265764431, -13.65522559108275935, 223.9268223389925083 ) ) ;
#24032=CARTESIAN_POINT ( 'NONE',  ( -0.2766206855629021466, -12.09920926763397553, 232.0000002394077399 ) ) ;
#24041=CARTESIAN_POINT ( 'NONE',  ( 24.60092358069999818, -12.94742893949999818, 225.2083619149999834 ) ) ;
#24068=CARTESIAN_POINT ( 'NONE',  ( 20.50716141039999840, 18.79636021840000026, 225.9999999149999894 ) ) ;
#24124=CARTESIAN_POINT ( 'NONE',  ( 23.69119887989999995, 20.94188554249999967, 222.0000000000000000 ) ) ;
#24139=CARTESIAN_POINT ( 'NONE',  ( 23.51173842660000091, 14.86483492350000013, 222.0000000000000000 ) ) ;
#24143=CARTESIAN_POINT ( 'NONE',  ( 26.80907646719999704, 9.389153233520001862, 229.0000000000000000 ) ) ;
#24145=ORIENTED_EDGE ( 'NONE', *, *, #16155, .F. ) ;
#24152=CARTESIAN_POINT ( 'NONE',  ( 26.80000000000000071, -6.394884621839999216E-14, 230.6999999999999886 ) ) ;
#24171=CARTESIAN_POINT ( 'NONE',  ( -11.74965333179999938, 3.618560759109999747, 232.6627643349999914 ) ) ;
#24172=CARTESIAN_POINT ( 'NONE',  ( -19.80526803549999926, 19.50877411520000138, 224.8000000000000114 ) ) ;
#24181=VECTOR ( 'NONE', #21637, 1000.000000000000000 ) ;
#24189=FACE_OUTER_BOUND ( 'NONE', #31046, .T. ) ;
#24192=EDGE_LOOP ( 'NONE', ( #1807, #18792, #30887, #12257 ) ) ;
#24200=CARTESIAN_POINT ( 'NONE',  ( 9.657736559230000850, -7.680833809369999265, 232.6627648150000027 ) ) ;
#24211=CARTESIAN_POINT ( 'NONE',  ( -24.58975347950000057, -12.96948186770000078, 224.6893543200000067 ) ) ;
#24242=EDGE_CURVE ( 'NONE', #18572, #979, #3673, .T. ) ;
#24265=B_SPLINE_SURFACE_WITH_KNOTS ( 'NONE', 5, 5, ( 
 ( #28513, #14628, #627, #12563, #13890, #14776, #25857, #9900, #12251 ),
 ( #18603, #30883, #22024, #2090, #11680, #22169, #9313, #28200, #29090 ),
 ( #24378, #21871, #2971, #319, #2816, #28358, #7536, #17128, #4295 ),
 ( #11528, #12408, #477, #10059, #19655, #29238, #7678, #17280, #26890 ),
 ( #5329, #14933, #21130, #9153, #24530, #18757, #6803, #10666, #24682 ),
 ( #22323, #15086, #29396, #20261, #15232, #8135, #15388, #776, #12876 ) ),
 .UNSPECIFIED., .F., .F., .F.,
 ( 6, 6 ),
 ( 6, 3, 6 ),
 ( 64.89339659379999148, 88.33140247330000250 ),
 ( 8.011061266649999624, 8.811732102769999742, 9.612402938880000747 ),
 .UNSPECIFIED. ) ;
#24291=CARTESIAN_POINT ( 'NONE',  ( 26.54997920389999777, 9.298361011320000813, 229.7313259189999712 ) ) ;
#24292=CARTESIAN_POINT ( 'NONE',  ( -6.408211168649999401, 17.12116672390000005, 230.6999999999999886 ) ) ;
#24326=CARTESIAN_POINT ( 'NONE',  ( -10.46518171449999990, 6.538123262210000064, 232.6627643349999914 ) ) ;
#24328=CARTESIAN_POINT ( 'NONE',  ( -8.359833048262370170, 8.751033796363188344, 232.0000000000050022 ) ) ;
#24334=CARTESIAN_POINT ( 'NONE',  ( -25.84755624059999946, 9.037785233839999322, 230.0000000000000000 ) ) ;
#24338=CARTESIAN_POINT ( 'NONE',  ( 11.95683611934412838, -1.871217229727538678, 232.0000002394077399 ) ) ;
#24344=CARTESIAN_POINT ( 'NONE',  ( 24.25004754381673422, -14.97293715294370031, 224.2649987588634417 ) ) ;
#24378=CARTESIAN_POINT ( 'NONE',  ( -23.94309786560000219, 13.28188914049999880, 230.0000000000000000 ) ) ;
#24394=CARTESIAN_POINT ( 'NONE',  ( 20.27681456348847178, 20.00004247328156026, 229.2644764541421125 ) ) ;
#24425=VERTEX_POINT ( 'NONE', #20653 ) ;
#24431=B_SPLINE_CURVE_WITH_KNOTS ( 'NONE', 5,
 ( #9103, #18703, #15713, #28152, #13360, #30197 ),
 .UNSPECIFIED., .F., .F.,
 ( 6, 6 ),
 ( -16.82733224740000111, 0.000000000000000000 ),
 .UNSPECIFIED. ) ;
#24448=CARTESIAN_POINT ( 'NONE',  ( 28.50000000000000000, 1.273924582309999984E-25, 222.0000000000000000 ) ) ;
#24453=CARTESIAN_POINT ( 'NONE',  ( 21.20256267760000313, 17.00023892710000339, 230.0000000000000000 ) ) ;
#24454=CARTESIAN_POINT ( 'NONE',  ( -17.67198296649999634, -4.679706496339999688, 230.6999999999999886 ) ) ;
#24472=DIRECTION ( 'NONE',  ( 1.000000000000000000, 0.000000000000000000, 0.000000000000000000 ) ) ;
#24477=CARTESIAN_POINT ( 'NONE',  ( 23.55447120710000064, 16.04539730700000177, 222.0000000000000000 ) ) ;
#24482=CARTESIAN_POINT ( 'NONE',  ( -0.8673174292429999266, -12.23557166350000003, 232.6627643349999914 ) ) ;
#24484=CARTESIAN_POINT ( 'NONE',  ( 24.07552309629999954, -13.90001137839999856, 223.9000014189999774 ) ) ;
#24496=CARTESIAN_POINT ( 'NONE',  ( -4.960227444680000097, -16.90556345619999945, 230.0904314459999966 ) ) ;
#24499=CARTESIAN_POINT ( 'NONE',  ( 24.60666743799999878, -12.93650359530000138, 225.0000014190000002 ) ) ;
#24520=B_SPLINE_CURVE_WITH_KNOTS ( 'NONE', 1,
 ( #20594, #30034 ),
 .UNSPECIFIED., .F., .F.,
 ( 2, 2 ),
 ( -2.555882182119999914E-06, 0.7000000000009999335 ),
 .UNSPECIFIED. ) ;
#24523=B_SPLINE_CURVE_WITH_KNOTS ( 'NONE', 5,
 ( #17875, #27479, #15525, #4046, #20409, #29997, #3567, #11128, #18030 ),
 .UNSPECIFIED., .F., .F.,
 ( 6, 3, 6 ),
 ( 8.011061266649999624, 9.405960541640000727, 10.80085981660000094 ),
 .UNSPECIFIED. ) ;
#24525=CARTESIAN_POINT ( 'NONE',  ( -23.50695179570000093, -14.84192241259999889, 225.0000014190000002 ) ) ;
#24530=CARTESIAN_POINT ( 'NONE',  ( -27.53132592989999949, 4.642205353319999617, 229.7313259299999686 ) ) ;
#24545=CARTESIAN_POINT ( 'NONE',  ( 20.06951727433725452, 19.99997495482045551, 229.7339536094710581 ) ) ;
#24555=CARTESIAN_POINT ( 'NONE',  ( -23.93396852079376202, -14.14368280436500491, 223.9267465465173927 ) ) ;
#24568=B_SPLINE_CURVE_WITH_KNOTS ( 'NONE', 3,
 ( #19371, #29575, #24555, #29263, #19838, #2836, #9766, #21896, #17149, #26915, #22048, #12280 ),
 .UNSPECIFIED., .F., .F.,
 ( 4, 2, 2, 2, 2, 4 ),
 ( 0.000000000000000000, 0.2500000000000155986, 0.5000000000000311973, 0.6250000000000234257, 0.7500000000000156541, 1.000000000000000000 ),
 .UNSPECIFIED. ) ;
#24584=CARTESIAN_POINT ( 'NONE',  ( 25.32889099250000342, 14.06639286550000101, 229.7625741969999922 ) ) ;
#24606=CARTESIAN_POINT ( 'NONE',  ( 18.48841959639999644, 20.72769515089999715, 229.2930775960000176 ) ) ;
#24626=ORIENTED_EDGE ( 'NONE', *, *, #30030, .T. ) ;
#24633=CARTESIAN_POINT ( 'NONE',  ( -12.05432023370000039, -0.5681652772719999467, 231.9999989789999972 ) ) ;
#24635=CARTESIAN_POINT ( 'NONE',  ( 23.50667118420000179, -14.84174322970000048, 225.0000014190000002 ) ) ;
#24641=CARTESIAN_POINT ( 'NONE',  ( -26.80000000000000071, 4.518892556989999143, 230.0000000000000000 ) ) ;
#24663=CARTESIAN_POINT ( 'NONE',  ( 4.414854054520000126, 11.17832006019999902, 231.9999991140000191 ) ) ;
#24674=DIRECTION ( 'NONE',  ( -0.4353787270609792981, -0.9002473904559574747, 0.000000000000000000 ) ) ;
#24681=CARTESIAN_POINT ( 'NONE',  ( -19.55772779817724683, 19.99999847704128797, 230.2366316984319781 ) ) ;
#24682=CARTESIAN_POINT ( 'NONE',  ( -27.79999999980000069, 4.687507935210000198, 229.0000000000000000 ) ) ;
#24713=CARTESIAN_POINT ( 'NONE',  ( -1.419173393160000125E-06, -27.80022181310000207, 226.1000014189999945 ) ) ;
#24718=CARTESIAN_POINT ( 'NONE',  ( 1.089891362619999970, -28.47934442809999922, 224.6898179359999972 ) ) ;
#24739=CARTESIAN_POINT ( 'NONE',  ( -19.80526803560000104, 19.50877411510000314, 227.0000000000000000 ) ) ;
#24744=CARTESIAN_POINT ( 'NONE',  ( 24.48837202150000181, -14.58033361329999877, 223.9575292099999899 ) ) ;
#24747=CARTESIAN_POINT ( 'NONE',  ( -0.1472904996853126869, -28.50022958377793358, 223.9000014189999774 ) ) ;
#24751=CARTESIAN_POINT ( 'NONE',  ( -18.97091445539999910, 21.26865671770000077, 229.2404163060000144 ) ) ;
#24753=B_SPLINE_CURVE_WITH_KNOTS ( 'NONE', 1,
 ( #4752, #16231 ),
 .UNSPECIFIED., .F., .F.,
 ( 2, 2 ),
 ( -0.7031447686210000603, 1.118726812310288921E-05 ),
 .UNSPECIFIED. ) ;
#24755=CARTESIAN_POINT ( 'NONE',  ( 21.92823313370000093, 17.58202518589999741, 229.4485716779999791 ) ) ;
#24775=CARTESIAN_POINT ( 'NONE',  ( -13.61743661210000056, -27.34210457880000078, 229.7313233489999789 ) ) ;
#24778=B_SPLINE_CURVE_WITH_KNOTS ( 'NONE', 3,
 ( #4913, #6810, #2094, #16406 ),
 .UNSPECIFIED., .F., .F.,
 ( 4, 4 ),
 ( 0.000000000000000000, 1.000000000000000000 ),
 .UNSPECIFIED. ) ;
#24800=CARTESIAN_POINT ( 'NONE',  ( 7.366762595500000241E-07, 20.00000000000000000, 230.6999999999999886 ) ) ;
#24808=EDGE_CURVE ( 'NONE', #23376, #12887, #28433, .T. ) ;
#24812=ORIENTED_EDGE ( 'NONE', *, *, #4611, .F. ) ;
#24837=CARTESIAN_POINT ( 'NONE',  ( -19.20323824044135463, 20.00026142946846264, 230.4259854455875995 ) ) ;
#24838=CARTESIAN_POINT ( 'NONE',  ( 2.131628207279999844E-14, 1.421085471519999843E-14, 230.0904314459999966 ) ) ;
#24859=FACE_OUTER_BOUND ( 'NONE', #9271, .T. ) ;
#24891=ORIENTED_EDGE ( 'NONE', *, *, #18050, .T. ) ;
#24898=CARTESIAN_POINT ( 'NONE',  ( -3.441895295100000141, -11.73074823080000151, 232.6627637660000119 ) ) ;
#24899=FACE_OUTER_BOUND ( 'NONE', #8450, .T. ) ;
#24904=CARTESIAN_POINT ( 'NONE',  ( 24.62873585949999722, -14.34148440729999940, 223.9040349389999847 ) ) ;
#24907=CARTESIAN_POINT ( 'NONE',  ( -1.007063440337249816, -28.48249027448747839, 224.5017099588716007 ) ) ;
#24936=ORIENTED_EDGE ( 'NONE', *, *, #2788, .T. ) ;
#24943=CARTESIAN_POINT ( 'NONE',  ( 23.66291322330000213, -14.59162663150000050, 224.2398658380000143 ) ) ;
#24985=CARTESIAN_POINT ( 'NONE',  ( -19.14227085988751043, 20.00032846726916347, 230.4526156311602847 ) ) ;
#24996=VERTEX_POINT ( 'NONE', #7535 ) ;
#25003=DIRECTION ( 'NONE',  ( 0.000000000000000000, 0.000000000000000000, 1.000000000000000000 ) ) ;
#25020=CARTESIAN_POINT ( 'NONE',  ( 0.4702670923949999748, -27.79645255899999867, 226.0025203910000187 ) ) ;
#25042=CARTESIAN_POINT ( 'NONE',  ( 28.04325408099999706, 4.735556750389999792, 230.2432540810000319 ) ) ;
#25046=CARTESIAN_POINT ( 'NONE',  ( -28.50000000000000000, 1.776356839399999922E-14, 222.0000000000000000 ) ) ;
#25047=CARTESIAN_POINT ( 'NONE',  ( -20.30396346370000060, 20.00000000000000000, 228.5999999999999943 ) ) ;
#25058=CARTESIAN_POINT ( 'NONE',  ( 25.22625794089999829, -13.26224522399999906, 225.0000014190000002 ) ) ;
#25059=CARTESIAN_POINT ( 'NONE',  ( -21.20818545079999851, 16.99505982179999819, 230.6999999999999886 ) ) ;
#25063=CARTESIAN_POINT ( 'NONE',  ( 27.79999999999999716, 2.344791028010000161E-11, 222.0000000000000000 ) ) ;
#25064=CARTESIAN_POINT ( 'NONE',  ( -26.80000000069999899, -2.537339890029999712, 230.6999999999999886 ) ) ;
#25066=ORIENTED_EDGE ( 'NONE', *, *, #14214, .F. ) ;
#25097=CARTESIAN_POINT ( 'NONE',  ( 24.19477113890000197, -13.69187437440000110, 223.9201473980000117 ) ) ;
#25099=CARTESIAN_POINT ( 'NONE',  ( -14.09657507470000226, -28.30410041510000241, 222.0000000000000000 ) ) ;
#25108=CARTESIAN_POINT ( 'NONE',  ( 27.79999999990000248, 4.333901782529999025, 224.8000000000000114 ) ) ;
#25117=ORIENTED_EDGE ( 'NONE', *, *, #13303, .F. ) ;
#25118=CARTESIAN_POINT ( 'NONE',  ( 17.91270342211725008, 20.00000026367296968, 230.7000000000000739 ) ) ;
#25135=CARTESIAN_POINT ( 'NONE',  ( 19.80538173989999962, 19.50875420239999869, 228.5999999789999890 ) ) ;
#25137=CARTESIAN_POINT ( 'NONE',  ( 0.2820261973285071999, -27.79909623906206662, 223.9267880206792540 ) ) ;
#25142=CARTESIAN_POINT ( 'NONE',  ( -20.04009859691944584, 19.99997709909766641, 229.7758549911204398 ) ) ;
#25162=CARTESIAN_POINT ( 'NONE',  ( -27.79999999999999716, -2.354383354940000152E-11, 222.0000000000000000 ) ) ;
#25175=CARTESIAN_POINT ( 'NONE',  ( 0.07063658732340000190, -28.50016343120000073, 226.0986540789999992 ) ) ;
#25179=CARTESIAN_POINT ( 'NONE',  ( 0.03533597110129999691, -28.50021994999999819, 223.9000014189999774 ) ) ;
#25194=CARTESIAN_POINT ( 'NONE',  ( 24.38125476360000121, 13.54012337690000045, 230.6577119970000069 ) ) ;
#25197=CARTESIAN_POINT ( 'NONE',  ( 28.50000000000000000, 8.881784197000000993E-16, 222.0000000000000000 ) ) ;
#25203=ORIENTED_EDGE ( 'NONE', *, *, #7674, .F. ) ;
#25213=CARTESIAN_POINT ( 'NONE',  ( -26.58302938879999999, 9.294948734580000149, 230.5592437530000041 ) ) ;
#25216=EDGE_CURVE ( 'NONE', #10061, #29716, #19404, .T. ) ;
#25219=CARTESIAN_POINT ( 'NONE',  ( -19.80526803560000104, 19.50877411510000314, 228.1999999999999886 ) ) ;
#25242=B_SPLINE_CURVE_WITH_KNOTS ( 'NONE', 5,
 ( #25162, #23128, #25482, #20279, #18063, #6114, #13042, #30033, #13355 ),
 .UNSPECIFIED., .F., .F.,
 ( 6, 3, 6 ),
 ( 0.000000000000000000, 53.95537973340000093, 92.42745556099998794 ),
 .UNSPECIFIED. ) ;
#25255=CARTESIAN_POINT ( 'NONE',  ( 25.22625794089999829, -13.26224522399999906, 224.8958210039999983 ) ) ;
#25257=CARTESIAN_POINT ( 'NONE',  ( 26.05511440539999768, -14.93230011240000010, 229.0000000000000000 ) ) ;
#25265=CARTESIAN_POINT ( 'NONE',  ( 22.83442928010000017, 16.43389279790000046, 224.8000000000000114 ) ) ;
#25275=CARTESIAN_POINT ( 'NONE',  ( 20.19118761472760326, 19.99999729016618133, 229.5203474167158504 ) ) ;
#25276=EDGE_CURVE ( 'NONE', #30960, #4760, #6777, .T. ) ;
#25283=CARTESIAN_POINT ( 'NONE',  ( 26.05511440539999768, -14.93230011240000010, 229.0000000000000000 ) ) ;
#25287=DIRECTION ( 'NONE',  ( 1.000000000000000000, 0.000000000000000000, 0.000000000000000000 ) ) ;
#25295=( GEOMETRIC_REPRESENTATION_CONTEXT ( 3 ) GLOBAL_UNCERTAINTY_ASSIGNED_CONTEXT ( ( #12825 ) ) GLOBAL_UNIT_ASSIGNED_CONTEXT ( ( #3705, #1357, #30302 ) ) REPRESENTATION_CONTEXT ( 'NONE', 'WORKASPACE' ) );
#25309=ORIENTED_EDGE ( 'NONE', *, *, #25216, .F. ) ;
#25317=ORIENTED_EDGE ( 'NONE', *, *, #11164, .T. ) ;
#25326=CARTESIAN_POINT ( 'NONE',  ( -1.419173372180000084E-06, -27.80022181310000207, 223.9000014189999774 ) ) ;
#25330=DIRECTION ( 'NONE',  ( 0.2815395311429196301, 0.9595496299847262600, 0.000000000000000000 ) ) ;
#25332=CARTESIAN_POINT ( 'NONE',  ( -24.14787428015092274, -13.77541660134580326, 226.1000014189999376 ) ) ;
#25339=CARTESIAN_POINT ( 'NONE',  ( 19.80538173989999962, 19.50875420239999869, 227.3999999149999951 ) ) ;
#25344=EDGE_CURVE ( 'NONE', #13298, #28330, #631, .T. ) ;
#25356=ORIENTED_EDGE ( 'NONE', *, *, #19819, .T. ) ;
#25357=CARTESIAN_POINT ( 'NONE',  ( 18.34692404780000174, 20.56908522520000204, 230.5592437530000041 ) ) ;
#25361=CARTESIAN_POINT ( 'NONE',  ( -24.09302906149999757, -13.87041066189999938, 226.1000014189999945 ) ) ;
#25379=CARTESIAN_POINT ( 'NONE',  ( -27.04662643769999875, 9.457048792620000199, 230.2432540810000319 ) ) ;
#25381=CARTESIAN_POINT ( 'NONE',  ( -24.68204616399999907, -14.25020164319999871, 226.1000014189999945 ) ) ;
#25393=CARTESIAN_POINT ( 'NONE',  ( 23.55447120710000064, 16.04539730700000177, 222.0000000000000000 ) ) ;
#25395=ORIENTED_EDGE ( 'NONE', *, *, #22969, .F. ) ;
#25407=CARTESIAN_POINT ( 'NONE',  ( -27.24857305700000154, -10.01116691310000029, 229.9172022069999741 ) ) ;
#25409=CARTESIAN_POINT ( 'NONE',  ( -20.30396346370000060, 20.00000000000000000, 227.0000000000000000 ) ) ;
#25433=CARTESIAN_POINT ( 'NONE',  ( 22.83442928010000017, 16.43389279790000046, 223.3999999999999773 ) ) ;
#25439=CARTESIAN_POINT ( 'NONE',  ( -9.961462390591020011, -7.265484932597956913, 232.6627637660201628 ) ) ;
#25446=CARTESIAN_POINT ( 'NONE',  ( 24.64642659020000082, -14.31106159850000026, 226.0986569330000293 ) ) ;
#25456=CARTESIAN_POINT ( 'NONE',  ( -1.419173393149999842E-06, -27.80022181310000207, 226.1000014189999945 ) ) ;
#25457=DIRECTION ( 'NONE',  ( 1.000000000000000000, 0.000000000000000000, 0.000000000000000000 ) ) ;
#25459=CARTESIAN_POINT ( 'NONE',  ( 19.80538173989999962, 19.50875420239999869, 228.1999999569999886 ) ) ;
#25462=CARTESIAN_POINT ( 'NONE',  ( 0.9498610579744216631, -27.78396626330503594, 224.4416736066579858 ) ) ;
#25482=CARTESIAN_POINT ( 'NONE',  ( -23.10935684540000068, -20.42749692129999772, 222.0000000000000000 ) ) ;
#25493=CARTESIAN_POINT ( 'NONE',  ( 0.2402089773159999941, -27.79941220630000132, 223.9202078600000050 ) ) ;
#25507=CARTESIAN_POINT ( 'NONE',  ( -25.11765555659999904, -13.46780168200000105, 224.3191686030000369 ) ) ;
#25516=CARTESIAN_POINT ( 'NONE',  ( 18.97091807949999875, 21.26865672099999927, 229.0000000000000000 ) ) ;
#25524=CARTESIAN_POINT ( 'NONE',  ( -1.127665019380000189, -28.47796022459999676, 225.1040592169999854 ) ) ;
#25525=VERTEX_POINT ( 'NONE', #21283 ) ;
#25547=DIRECTION ( 'NONE',  ( 0.000000000000000000, 0.000000000000000000, 1.000000000000000000 ) ) ;
#25548=LINE ( 'NONE', #27734, #8241 ) ;
#25560=CARTESIAN_POINT ( 'NONE',  ( 26.94142135619999934, -7.057848136739999667, 230.0000000000000000 ) ) ;
#25564=EDGE_LOOP ( 'NONE', ( #5176, #11911, #14208, #14256 ) ) ;
#25584=CARTESIAN_POINT ( 'NONE',  ( -28.50000000000000000, 5.427757009279999762E-15, 222.0000000000000000 ) ) ;
#25592=( NAMED_UNIT ( * ) SI_UNIT ( $, .STERADIAN. ) SOLID_ANGLE_UNIT ( ) );
#25618=CARTESIAN_POINT ( 'NONE',  ( -24.09883371379999772, -15.21565466309999870, 225.0000014190000002 ) ) ;
#25619=CARTESIAN_POINT ( 'NONE',  ( 19.80538173169999894, 19.50875421069999760, 226.9999998930000231 ) ) ;
#25646=CARTESIAN_POINT ( 'NONE',  ( 5.548090509119999680, -11.02205857200000061, 232.6627648150000027 ) ) ;
#25647=DIRECTION ( 'NONE',  ( 0.000000000000000000, 0.000000000000000000, 1.000000000000000000 ) ) ;
#25650=CARTESIAN_POINT ( 'NONE',  ( -14.09657507470000226, -28.30410041680000077, 229.2404163060000144 ) ) ;
#25674=CARTESIAN_POINT ( 'NONE',  ( 18.97091807949999875, 21.26865672150000108, 229.2404163060000144 ) ) ;
#25677=CARTESIAN_POINT ( 'NONE',  ( -24.71725143720000162, -14.18911829940000047, 226.0986578700000109 ) ) ;
#25708=CARTESIAN_POINT ( 'NONE',  ( 22.36196472700000015, 17.71394650440000262, 223.9999999570000000 ) ) ;
#25720=CARTESIAN_POINT ( 'NONE',  ( 24.76888645009999834, -14.19515663950000040, 229.9751246520000052 ) ) ;
#25731=CARTESIAN_POINT ( 'NONE',  ( 28.50000000000000000, 7.746889549609999817E-15, 229.0000000000000000 ) ) ;
#25739=EDGE_CURVE ( 'NONE', #13739, #14446, #8645, .T. ) ;
#25748=SURFACE_SIDE_STYLE ('',( #20705 ) ) ;
#25768=CARTESIAN_POINT ( 'NONE',  ( 24.22190007760000086, -15.01852807150000046, 225.6806946080000102 ) ) ;
#25772=CARTESIAN_POINT ( 'NONE',  ( -1.115050571030000048, -28.47845913019999742, 225.2081166120000262 ) ) ;
#25803=CARTESIAN_POINT ( 'NONE',  ( -13.63290864800000080, -27.37311817530000013, 230.5592437530000041 ) ) ;
#25821=CARTESIAN_POINT ( 'NONE',  ( 3.550686847520000117E-05, -28.50022181210000127, 223.9000014189999774 ) ) ;
#25830=CARTESIAN_POINT ( 'NONE',  ( -1.127665019380000189, -28.47796022459999676, 225.0000014190000002 ) ) ;
#25832=CARTESIAN_POINT ( 'NONE',  ( -25.22658730140000216, -13.26242337740000110, 225.0000014190000002 ) ) ;
#25840=CARTESIAN_POINT ( 'NONE',  ( -18.31101975560000028, 19.88193351600000014, 229.9783743860000129 ) ) ;
#25850=CARTESIAN_POINT ( 'NONE',  ( -24.25909092270000045, -14.95913241679999928, 225.7602679599999931 ) ) ;
#25851=CARTESIAN_POINT ( 'NONE',  ( 27.24857305730000334, 4.340180672490000177E-12, 229.9172022069999741 ) ) ;
#25857=CARTESIAN_POINT ( 'NONE',  ( -18.48840241599999956, 20.72770724009999910, 229.2930776200000196 ) ) ;
#25868=COLOUR_RGB ( '', 0.40784314, 0.44705882, 0.49803922) ;
#25877=CARTESIAN_POINT ( 'NONE',  ( 20.64716981400000151, -20.77933506639999806, 229.1414209110000115 ) ) ;
#25886=CARTESIAN_POINT ( 'NONE',  ( 11.98357239787091189, 2.900346313630838058, 232.6627636033630324 ) ) ;
#25891=CARTESIAN_POINT ( 'NONE',  ( -22.97554860800000043, 15.65134970540000126, 222.0000000000000000 ) ) ;
#25892=CARTESIAN_POINT ( 'NONE',  ( 0.8959394325450000807, -28.48619164239999790, 225.6801530179999986 ) ) ;
#25902=TOROIDAL_SURFACE ( 'NONE', #22853, 18.16530045470000232, 1.699999999999999956 ) ;
#25907=CARTESIAN_POINT ( 'NONE',  ( 1.906343942476213638, 12.18129127136987400, 232.6627637660202481 ) ) ;
#25924=CARTESIAN_POINT ( 'NONE',  ( 17.83931934289999788, 20.00000000000000000, 230.7000122960000112 ) ) ;
#25925=CARTESIAN_POINT ( 'NONE',  ( -27.79999999999999716, -2.355677988119999702E-11, 223.3999999999999773 ) ) ;
#25927=CARTESIAN_POINT ( 'NONE',  ( -0.8057362887179999600, -27.78873281830000153, 225.7596419580000315 ) ) ;
#25931=CARTESIAN_POINT ( 'NONE',  ( 19.80538173169999894, 19.50875421069999760, 226.9999998930000231 ) ) ;
#25949=CARTESIAN_POINT ( 'NONE',  ( -5.260974094009999824, -10.78653348610000151, 231.9999991140000191 ) ) ;
#25953=CARTESIAN_POINT ( 'NONE',  ( -23.65604620319999896, -20.91081238350000149, 229.4982322489999831 ) ) ;
#25955=CARTESIAN_POINT ( 'NONE',  ( -24.22223838309999877, -15.01863363600000056, 224.3191706570000292 ) ) ;
#25961=CARTESIAN_POINT ( 'NONE',  ( -24.19505510210000310, -13.69211658319999891, 223.9201349309999785 ) ) ;
#25984=CARTESIAN_POINT ( 'NONE',  ( -24.80426825129999813, -14.03688870149999879, 226.0798679069999935 ) ) ;
#25985=CARTESIAN_POINT ( 'NONE',  ( -24.60699806910000120, -12.93667933180000063, 225.0000014190000002 ) ) ;
#25991=CARTESIAN_POINT ( 'NONE',  ( -20.30397143389999925, 20.00000785070000120, 229.1256643320000137 ) ) ;
#25999=CARTESIAN_POINT ( 'NONE',  ( -24.02415253779999915, -13.98938335050000070, 226.0959707279999975 ) ) ;
#26029=CARTESIAN_POINT ( 'NONE',  ( 8.673459918069999830, -27.31266770540000266, 222.0000000000000000 ) ) ;
#26042=CARTESIAN_POINT ( 'NONE',  ( 1.099998580829999906, -27.77839262550000043, 225.0000014190000002 ) ) ;
#26075=EDGE_LOOP ( 'NONE', ( #20169, #2482, #11425, #17293 ) ) ;
#26077=CARTESIAN_POINT ( 'NONE',  ( 24.25874038310000103, -14.95904359230000047, 225.7601370010000039 ) ) ;
#26078=CARTESIAN_POINT ( 'NONE',  ( 19.68705805829999989, 19.53816415229999848, 229.3697640839999963 ) ) ;
#26079=CARTESIAN_POINT ( 'NONE',  ( -27.79999999990000248, 4.328052761030000362, 226.2000000000000171 ) ) ;
#26081=CARTESIAN_POINT ( 'NONE',  ( -0.2462327729630000017, -28.49941772390000239, 226.0797932899999978 ) ) ;
#26092=CARTESIAN_POINT ( 'NONE',  ( -24.22223838309999877, -15.01863363600000056, 224.3191706570000292 ) ) ;
#26104=CARTESIAN_POINT ( 'NONE',  ( -3.934873304249999482, -11.62798211380000168, 232.6627648150000027 ) ) ;
#26108=CARTESIAN_POINT ( 'NONE',  ( 20.27449537109999866, -20.40427436439999909, 230.6577119970000069 ) ) ;
#26110=CARTESIAN_POINT ( 'NONE',  ( -24.48873108240000107, -14.58042505439999914, 223.9574921880000034 ) ) ;
#26146=CARTESIAN_POINT ( 'NONE',  ( -20.28767293760000001, 20.00000794000000326, 229.2539848859999836 ) ) ;
#26175=CARTESIAN_POINT ( 'NONE',  ( 27.71720220739999974, 1.975664076780000201E-11, 229.4485730569999760 ) ) ;
#26176=CARTESIAN_POINT ( 'NONE',  ( 24.60666973299078109, -12.93650480179403139, 225.0734590689982610 ) ) ;
#26177=CARTESIAN_POINT ( 'NONE',  ( 27.70209893939999901, -2.554094161149999653, 222.0000000000000000 ) ) ;
#26185=CARTESIAN_POINT ( 'NONE',  ( -13.75032424529999986, -27.60893268180000248, 229.0000000050000040 ) ) ;
#26190=CARTESIAN_POINT ( 'NONE',  ( -24.09883371379999772, -15.21565466309999870, 225.0000014190000002 ) ) ;
#26191=CARTESIAN_POINT ( 'NONE',  ( -24.50617912300000256, 13.34342669039999940, 222.0000000000000000 ) ) ;
#26208=CARTESIAN_POINT ( 'NONE',  ( -12.18129127137019907, 1.906343942474053366, 232.6627637660202197 ) ) ;
#26217=CARTESIAN_POINT ( 'NONE',  ( 24.25874038310000103, -14.95904359230000047, 224.2398658380000143 ) ) ;
#26223=CARTESIAN_POINT ( 'NONE',  ( 24.11883219139999923, -15.18335225210000061, 225.3105549429999996 ) ) ;
#26224=CARTESIAN_POINT ( 'NONE',  ( 20.28774895549999968, 20.00000871369999800, 229.2541281029999993 ) ) ;
#26228=CARTESIAN_POINT ( 'NONE',  ( -1.419173379759999885E-06, -27.80022181310000207, 226.1000014189999945 ) ) ;
#26233=CARTESIAN_POINT ( 'NONE',  ( 23.50667118420000179, -14.84174322970000048, 225.0000014190000002 ) ) ;
#26234=CARTESIAN_POINT ( 'NONE',  ( 4.885731121091885676, 11.07235364852818549, 232.0000002394077967 ) ) ;
#26254=CARTESIAN_POINT ( 'NONE',  ( -2.753981004559999946, -11.98181634260000017, 232.6627648150000027 ) ) ;
#26259=CARTESIAN_POINT ( 'NONE',  ( -22.69220507780000062, -20.05882317629999889, 230.6577119970000069 ) ) ;
#26285=CARTESIAN_POINT ( 'NONE',  ( -0.03443693864410000277, -27.80022362959999782, 223.9000014189999774 ) ) ;
#26295=CARTESIAN_POINT ( 'NONE',  ( -19.80526744929999694, 19.50877353739999975, 229.0739196179999908 ) ) ;
#26303=CARTESIAN_POINT ( 'NONE',  ( -27.79999999999999716, -2.360778239559999931E-11, 229.0000000000000000 ) ) ;
#26322=EDGE_LOOP ( 'NONE', ( #27295, #25066, #3065, #28779 ) ) ;
#26351=CARTESIAN_POINT ( 'NONE',  ( 26.80000000000000071, 3.197442310919999608E-14, 230.0000000000000000 ) ) ;
#26352=CARTESIAN_POINT ( 'NONE',  ( -16.30907199849999856, 8.426333778950001019, 230.6999999999999886 ) ) ;
#26365=CARTESIAN_POINT ( 'NONE',  ( 25.89948290199999903, 7.563190779290000165, 230.6999999999999886 ) ) ;
#26388=CARTESIAN_POINT ( 'NONE',  ( -22.83911268609999823, 16.42879705509999866, 224.8000000000000114 ) ) ;
#26396=CARTESIAN_POINT ( 'NONE',  ( -27.53132593009999951, -1.221706759790000127E-11, 229.7313259299999686 ) ) ;
#26401=ORIENTED_EDGE ( 'NONE', *, *, #19186, .T. ) ;
#26402=CARTESIAN_POINT ( 'NONE',  ( 25.17364887440000132, -13.36205984479999920, 225.5069763079999916 ) ) ;
#26417=CARTESIAN_POINT ( 'NONE',  ( 27.29823224869999976, -7.151321944500000249, 230.6577119970000069 ) ) ;
#26422=CARTESIAN_POINT ( 'NONE',  ( -0.8233448747507865484, -27.78811367915593777, 225.7327679764803179 ) ) ;
#26443=CARTESIAN_POINT ( 'NONE',  ( -0.06887222117169999880, -27.80017212539999960, 223.9013489249999793 ) ) ;
#26466=EDGE_LOOP ( 'NONE', ( #19554, #5671, #3725, #7356 ) ) ;
#26476=ORIENTED_EDGE ( 'NONE', *, *, #21008, .F. ) ;
#26481=ORIENTED_EDGE ( 'NONE', *, *, #22930, .T. ) ;
#26483=CARTESIAN_POINT ( 'NONE',  ( 3.378474373710000034, 11.51459555979999827, 232.0000000000000000 ) ) ;
#26523=CARTESIAN_POINT ( 'NONE',  ( 24.22190007760000086, -15.01852807150000046, 224.3193082299999901 ) ) ;
#26541=CARTESIAN_POINT ( 'NONE',  ( 23.52223098035388205, -14.81718486479981323, 225.2893105631158051 ) ) ;
#26549=CARTESIAN_POINT ( 'NONE',  ( 24.09856112909999837, -15.21545593799999985, 225.0000014190000002 ) ) ;
#26562=CARTESIAN_POINT ( 'NONE',  ( 12.10980759760000147, 2.370578709670000173, 232.6627648150000027 ) ) ;
#26565=CARTESIAN_POINT ( 'NONE',  ( 28.35924375230000294, -7.429275285240000137, 229.7625741969999922 ) ) ;
#26571=CARTESIAN_POINT ( 'NONE',  ( -0.5500250885004874801, -27.79512802401430704, 225.9640385793438497 ) ) ;
#26575=CARTESIAN_POINT ( 'NONE',  ( 21.81274943930000276, 17.27884304029999640, 223.9999999570000000 ) ) ;
#26586=EDGE_CURVE ( 'NONE', #15092, #6979, #5787, .T. ) ;
#26590=VERTEX_POINT ( 'NONE', #24496 ) ;
#26596=ORIENTED_EDGE ( 'NONE', *, *, #10220, .T. ) ;
#26626=ORIENTED_EDGE ( 'NONE', *, *, #13520, .F. ) ;
#26689=CARTESIAN_POINT ( 'NONE',  ( 23.58655966524121794, -14.71450914371738605, 225.5583129603366785 ) ) ;
#26709=B_SPLINE_SURFACE_WITH_KNOTS ( 'NONE', 5, 5, ( 
 ( #23281, #23448, #4080, #11626, #7057, #21540, #30979, #4545, #13995 ),
 ( #16188, #30675, #11932, #9253, #18861, #4698, #23913, #21224, #15800 ),
 ( #16648, #1878, #26259, #28761, #28618, #30522, #25953, #30825, #9101 ),
 ( #28150, #18701, #23602, #25803, #13836, #4236, #28459, #25650, #20920 ),
 ( #2038, #21078, #11476, #28301, #6894, #6745, #16345, #16496, #2193 ),
 ( #4390, #1723, #26108, #14148, #23753, #11782, #21387, #9411, #19015 ),
 ( #14307, #2348, #13676, #9576, #19174, #7215, #11322, #8949, #18549 ),
 ( #6590, #22005, #26417, #2953, #10043, #26565, #27027, #306, #12238 ),
 ( #7821, #26875, #21855, #4859, #29381, #12086, #15070, #14460, #12547 ) ),
 .UNSPECIFIED., .F., .F., .F.,
 ( 6, 3, 6 ),
 ( 6, 3, 6 ),
 ( 0.000000000000000000, 54.03331039209999886, 92.56095350929999199 ),
 ( 8.011061266649999624, 9.405960541640000727, 10.80085981660000094 ),
 .UNSPECIFIED. ) ;
#26738=ORIENTED_EDGE ( 'NONE', *, *, #22969, .T. ) ;
#26744=CARTESIAN_POINT ( 'NONE',  ( -0.2462327729630000017, -28.49941772390000239, 223.9202095490000204 ) ) ;
#26768=EDGE_LOOP ( 'NONE', ( #4116, #5151, #26596, #16888, #1920 ) ) ;
#26795=CARTESIAN_POINT ( 'NONE',  ( -27.79999999970000246, -10.21376199200000201, 229.0000000000000000 ) ) ;
#26804=EDGE_CURVE ( 'NONE', #5832, #14789, #19284, .T. ) ;
#26806=CARTESIAN_POINT ( 'NONE',  ( 27.24857305720000156, 4.601362004630000335, 229.9172022069999741 ) ) ;
#26807=CARTESIAN_POINT ( 'NONE',  ( -3.184804871879999943, 18.07879523729999960, 230.6999999999999886 ) ) ;
#26827=B_SPLINE_CURVE_WITH_KNOTS ( 'NONE', 5,
 ( #15910, #11503, #3955, #16375, #9129, #8661 ),
 .UNSPECIFIED., .F., .F.,
 ( 6, 6 ),
 ( 76.96280491019999204, 81.23072221990000230 ),
 .UNSPECIFIED. ) ;
#26829=AXIS2_PLACEMENT_3D ( 'NONE', #15043, #1304, #27721 ) ;
#26836=CARTESIAN_POINT ( 'NONE',  ( -11.18209233740000208, 4.537649734730000439, 231.9999989789999972 ) ) ;
#26855=CARTESIAN_POINT ( 'NONE',  ( 25.22036945370000183, -13.27344566769999901, 225.2083619149999834 ) ) ;
#26869=CARTESIAN_POINT ( 'NONE',  ( -25.21256988278790701, -13.28918881462575285, 224.7093197384999428 ) ) ;
#26875=CARTESIAN_POINT ( 'NONE',  ( 27.04041630560000087, -5.329070518199999767E-14, 230.6999999999999886 ) ) ;
#26881=FACE_OUTER_BOUND ( 'NONE', #14448, .T. ) ;
#26885=CARTESIAN_POINT ( 'NONE',  ( 0.8233563490081640124, -27.78802870620434007, 224.2672522965996791 ) ) ;
#26890=CARTESIAN_POINT ( 'NONE',  ( -26.81201737230000148, 9.375055877159999440, 229.0000000000000000 ) ) ;
#26915=CARTESIAN_POINT ( 'NONE',  ( -23.52253596342320918, -14.81732487615617089, 224.7105397188568645 ) ) ;
#26942=EDGE_LOOP ( 'NONE', ( #21713, #1157, #21372, #21348, #2674 ) ) ;
#26944=CARTESIAN_POINT ( 'NONE',  ( 28.35924375240000117, 4.788916714149999088, 229.7625741969999922 ) ) ;
#26959=CARTESIAN_POINT ( 'NONE',  ( 28.23994777610000284, 4.869985548859999902, 222.0000000000000000 ) ) ;
#26963=CARTESIAN_POINT ( 'NONE',  ( 17.93345776099999966, 20.10553696510000066, 230.0000000000000000 ) ) ;
#26989=CARTESIAN_POINT ( 'NONE',  ( 7.908773014210000341, 16.35323874420000223, 230.6999999999999886 ) ) ;
#26995=CARTESIAN_POINT ( 'NONE',  ( 24.02382125689999981, -13.98923529139999999, 223.9040349389999847 ) ) ;
#27009=CARTESIAN_POINT ( 'NONE',  ( 24.09271802119999961, -13.87022289859999979, 226.1000014189999945 ) ) ;
#27010=EDGE_CURVE ( 'NONE', #18572, #15181, #12751, .T. ) ;
#27024=CARTESIAN_POINT ( 'NONE',  ( 9.479780402439999420, -7.539304615940000787, 231.9999991140000191 ) ) ;
#27027=CARTESIAN_POINT ( 'NONE',  ( 28.45771199700000054, -7.455071025909999705, 229.4982322489999831 ) ) ;
#27040=CARTESIAN_POINT ( 'NONE',  ( -19.39816331875209698, 20.00000148357435137, 230.3275357089658542 ) ) ;
#27056=CARTESIAN_POINT ( 'NONE',  ( 24.48837202150000181, -14.58033361329999877, 226.0424736289999714 ) ) ;
#27079=CARTESIAN_POINT ( 'NONE',  ( 0.3832430167609999772, -28.49789927060000139, 223.9576737099999946 ) ) ;
#27122=B_SPLINE_CURVE_WITH_KNOTS ( 'NONE', 5,
 ( #20722, #10652, #30157, #1061, #3407, #11125, #8277, #7971, #8429, #10816, #18190, #3724, #10505, #17871, #27476 ),
 .UNSPECIFIED., .F., .F.,
 ( 6, 3, 3, 3, 6 ),
 ( 0.000000000000000000, 0.1000000000028630903, 0.3999999999999999667, 0.7000000000005727196, 1.000000000000000000 ),
 .UNSPECIFIED. ) ;
#27135=CARTESIAN_POINT ( 'NONE',  ( -27.71720220739999974, 1.978861519090000090E-11, 229.4485730569999760 ) ) ;
#27145=CARTESIAN_POINT ( 'NONE',  ( 17.99586598600000187, 19.96083381589999917, 229.9999934530000019 ) ) ;
#27150=CARTESIAN_POINT ( 'NONE',  ( 23.50666810109999716, -14.84174128299999929, 224.8958160969999938 ) ) ;
#27175=CARTESIAN_POINT ( 'NONE',  ( -25.22658730140538808, -13.26242337740151811, 224.8524123125729943 ) ) ;
#27178=CARTESIAN_POINT ( 'NONE',  ( 1.423247168829999991E-05, 20.00000000000000000, 230.0000000010000178 ) ) ;
#27194=CARTESIAN_POINT ( 'NONE',  ( -18.40310945181386515, 20.00006322233851108, 230.6579732124013162 ) ) ;
#27214=CARTESIAN_POINT ( 'NONE',  ( -20.50698707569999968, 18.79638478329999884, 226.0000000000000000 ) ) ;
#27222=CARTESIAN_POINT ( 'NONE',  ( -24.21578250576721913, -13.65559031243956412, 226.0732541239276259 ) ) ;
#27240=ORIENTED_EDGE ( 'NONE', *, *, #19711, .T. ) ;
#27243=CARTESIAN_POINT ( 'NONE',  ( 28.45771199730000234, 2.371705317339999772E-14, 229.4982322489999831 ) ) ;
#27255=CARTESIAN_POINT ( 'NONE',  ( 23.88690489929999927, -14.22221811490000043, 223.9575292099999899 ) ) ;
#27259=CARTESIAN_POINT ( 'NONE',  ( -1.097519451206210750, -28.47920044965180608, 224.7095162403817312 ) ) ;
#27262=CARTESIAN_POINT ( 'NONE',  ( 24.80399018339999628, -14.03663607480000053, 223.9201473980000117 ) ) ;
#27263=CARTESIAN_POINT ( 'NONE',  ( -25.42409647459999888, 14.10343940200000112, 229.4982322489999831 ) ) ;
#27266=CARTESIAN_POINT ( 'NONE',  ( -19.80526803560000104, 19.50877411510000314, 227.3999999999999773 ) ) ;
#27295=ORIENTED_EDGE ( 'NONE', *, *, #29764, .F. ) ;
#27298=FACE_BOUND ( 'NONE', #16481, .T. ) ;
#27299=CARTESIAN_POINT ( 'NONE',  ( 24.04107748430000058, -13.95955969929999974, 223.9013459049999994 ) ) ;
#27307=CARTESIAN_POINT ( 'NONE',  ( -5.361385120500000490, 31.61859227569999931, 229.0000000000000000 ) ) ;
#27324=CIRCLE ( 'NONE', #26829, 18.16530045500000057 ) ;
#27345=CARTESIAN_POINT ( 'NONE',  ( -18.53535511557664961, 20.00004277161199440, 230.6343261903482187 ) ) ;
#27349=TOROIDAL_SURFACE ( 'NONE', #3224, 18.16530045470000232, 1.000000000000000000 ) ;
#27362=COLOUR_RGB ( '', 0.40784314, 0.44705882, 0.49803922) ;
#27364=DIRECTION ( 'NONE',  ( 0.4353787270609792981, 0.9002473904559574747, 0.000000000000000000 ) ) ;
#27379=CARTESIAN_POINT ( 'NONE',  ( -24.55259642772470130, -13.03965859083635515, 225.4961348835367971 ) ) ;
#27381=CARTESIAN_POINT ( 'NONE',  ( 24.68173674080000168, -14.25001227039999918, 226.1000014189999945 ) ) ;
#27386=ORIENTED_EDGE ( 'NONE', *, *, #24242, .T. ) ;
#27414=CARTESIAN_POINT ( 'NONE',  ( -18.87722060250000311, 21.16361474240000007, 229.7625741969999922 ) ) ;
#27416=CARTESIAN_POINT ( 'NONE',  ( 5.229687933660000176, -30.84198039109999812, 222.0000000000000000 ) ) ;
#27437=CARTESIAN_POINT ( 'NONE',  ( -27.09307779329999732, -9.954037724019999089, 229.9751247039999953 ) ) ;
#27445=CARTESIAN_POINT ( 'NONE',  ( 24.39498713390000262, -13.33204241800000034, 224.0987054560000047 ) ) ;
#27461=CARTESIAN_POINT ( 'NONE',  ( -25.22658730140000216, -13.26242337740000110, 225.0000014190000002 ) ) ;
#27467=CARTESIAN_POINT ( 'NONE',  ( 18.25326690153244513, 20.00000274250295718, 230.6772558227679042 ) ) ;
#27476=CARTESIAN_POINT ( 'NONE',  ( -1.100001419170000050, -27.77850706310000106, 225.0000014190000002 ) ) ;
#27479=CARTESIAN_POINT ( 'NONE',  ( 27.04041630560000087, -5.217841840389998853E-14, 230.6999999999999886 ) ) ;
#27513=EDGE_CURVE ( 'NONE', #5832, #10448, #24523, .T. ) ;
#27525=CARTESIAN_POINT ( 'NONE',  ( 0.3737937747469999850, -27.79795631750000240, 226.0423291289999952 ) ) ;
#27550=CARTESIAN_POINT ( 'NONE',  ( 26.80000000000000071, 4.525613202489999765, 230.6999999999999886 ) ) ;
#27557=CARTESIAN_POINT ( 'NONE',  ( -0.03526712872429999673, -28.50022367440000082, 226.1000014189999945 ) ) ;
#27563=CARTESIAN_POINT ( 'NONE',  ( -26.32808186270000306, 9.205804489829999326, 230.6577119970000069 ) ) ;
#27568=CARTESIAN_POINT ( 'NONE',  ( 21.73374413810000050, -15.98809491730000154, 230.6999999999999886 ) ) ;
#27577=ORIENTED_EDGE ( 'NONE', *, *, #21723, .F. ) ;
#27579=DIRECTION ( 'NONE',  ( -0.4353787270609792981, -0.9002473904559574747, 0.000000000000000000 ) ) ;
#27604=CARTESIAN_POINT ( 'NONE',  ( 25.22625794089999829, -13.26224522399999906, 225.0000014190000002 ) ) ;
#27611=VERTEX_POINT ( 'NONE', #21192 ) ;
#27613=CARTESIAN_POINT ( 'NONE',  ( 25.26809612939999994, 12.77001324749999966, 224.8000000000000114 ) ) ;
#27623=CARTESIAN_POINT ( 'NONE',  ( 20.08457158244946683, 19.99997717933547392, 229.7115254020307020 ) ) ;
#27628=FACE_OUTER_BOUND ( 'NONE', #25564, .T. ) ;
#27687=EDGE_CURVE ( 'NONE', #19467, #27946, #8331, .T. ) ;
#27700=CARTESIAN_POINT ( 'NONE',  ( -1.015151870899999809, -28.48229306780000059, 224.4935097720000101 ) ) ;
#27702=CARTESIAN_POINT ( 'NONE',  ( -24.39524108160000182, -13.33235248870000156, 225.9014032059999977 ) ) ;
#27709=CARTESIAN_POINT ( 'NONE',  ( 3.550686850769999806E-05, -28.50022181210000127, 226.1000014189999945 ) ) ;
#27715=CARTESIAN_POINT ( 'NONE',  ( 25.22625794089999829, -13.26224522399999906, 225.0000014190000002 ) ) ;
#27719=CARTESIAN_POINT ( 'NONE',  ( -27.56257419730000180, 4.647474305650000304, 230.5592437530000041 ) ) ;
#27721=DIRECTION ( 'NONE',  ( 1.000000000000000000, 0.000000000000000000, 0.000000000000000000 ) ) ;
#27722=CARTESIAN_POINT ( 'NONE',  ( -24.05864279069999867, -13.92996648929999992, 226.1000014189999945 ) ) ;
#27724=CARTESIAN_POINT ( 'NONE',  ( 20.64716981389999972, -20.77933506589999979, 222.0000000000000000 ) ) ;
#27725=CARTESIAN_POINT ( 'NONE',  ( 18.02779606829999892, 3.032253802040000057, 230.6999999999999886 ) ) ;
#27733=CARTESIAN_POINT ( 'NONE',  ( -25.20890834729999952, -13.29605215849999844, 225.3106485179999936 ) ) ;
#27734=CARTESIAN_POINT ( 'NONE',  ( 133283.2115610000037, 454258.9661130000022, -160669.8390839999774 ) ) ;
#27742=B_SPLINE_CURVE_WITH_KNOTS ( 'NONE', 3,
 ( #20088, #20393, #20547, #6223, #25439, #18963, #11727, #23550, #26208, #28097, #16135, #6538, #4342, #28247, #13461, #18803, #25907, #13779 ),
 .UNSPECIFIED., .F., .F.,
 ( 4, 2, 2, 2, 2, 2, 2, 2, 4 ),
 ( 0.000000000000000000, 0.1249999999999999722, 0.2500000000000000000, 0.3750000000000000000, 0.5000000000000001110, 0.6250000000000001110, 0.7500000000000000000, 0.8750000000000000000, 1.000000000000000000 ),
 .UNSPECIFIED. ) ;
#27751=DIRECTION ( 'NONE',  ( 1.000000000000000000, 0.000000000000000000, 0.000000000000000000 ) ) ;
#27757=B_SPLINE_CURVE_WITH_KNOTS ( 'NONE', 5,
 ( #11685, #23810, #9477, #21750, #9158, #200, #31040, #14369, #23967, #19231, #28815, #9792, #19392, #28981, #7424 ),
 .UNSPECIFIED., .F., .F.,
 ( 6, 3, 3, 3, 6 ),
 ( 0.000000000000000000, 0.2999999999999999889, 0.6000000000034357850, 0.8999999999965643260, 1.000000000000000000 ),
 .UNSPECIFIED. ) ;
#27771=CARTESIAN_POINT ( 'NONE',  ( 22.83442928010000017, 16.43389279790000046, 229.0000000000000000 ) ) ;
#27779=B_SPLINE_CURVE_WITH_KNOTS ( 'NONE', 5,
 ( #13246, #25064, #22701, #5855, #13407, #17654, #30094, #3497, #6170, #10590, #8520, #11059, #22863, #11209, #3821, #15770, #1307, #27568, #13093, #18122, #10901, #23022, #1468, #3339 ),
 .UNSPECIFIED., .F., .F.,
 ( 6, 3, 3, 3, 3, 3, 3, 6 ),
 ( 0.000000000000000000, 18.45572787860000119, 36.93774665009999580, 55.41656326359999696, 72.02514973920000330, 90.47575867250000670, 108.9324419860000006, 122.5879169570000045 ),
 .UNSPECIFIED. ) ;
#27782=CARTESIAN_POINT ( 'NONE',  ( 18.40063513716208377, 20.00005172663331976, 230.6578942932893597 ) ) ;
#27784=CARTESIAN_POINT ( 'NONE',  ( -18.62349881349999947, 19.80369232029999793, 229.9327143820000003 ) ) ;
#27786=CARTESIAN_POINT ( 'NONE',  ( 24.04107748419999879, -13.95955969929999974, 226.0986569330000293 ) ) ;
#27801=CARTESIAN_POINT ( 'NONE',  ( 1.063741597852546183, -27.77980805031950240, 225.2880308456763885 ) ) ;
#27803=CARTESIAN_POINT ( 'NONE',  ( -24.62906106470000012, -14.34164290000000008, 226.0959707279999975 ) ) ;
#27839=CARTESIAN_POINT ( 'NONE',  ( 0.6686231747119999458, -28.49266848160000265, 224.0990955869999937 ) ) ;
#27849=ORIENTED_EDGE ( 'NONE', *, *, #18694, .T. ) ;
#27854=EDGE_LOOP ( 'NONE', ( #2410, #16486, #23970, #2252 ) ) ;
#27864=CARTESIAN_POINT ( 'NONE',  ( 22.54750148980000191, 18.07861229659999935, 229.2404163060000144 ) ) ;
#27885=CARTESIAN_POINT ( 'NONE',  ( -27.04041630560000087, 4.559430447050000446, 230.6999999999999886 ) ) ;
#27889=CARTESIAN_POINT ( 'NONE',  ( 13.76031882590000066, 12.03543611500000132, 230.6999999999999886 ) ) ;
#27898=CARTESIAN_POINT ( 'NONE',  ( -25.17394274020000111, -13.36230406159999973, 225.5071265450000055 ) ) ;
#27914=CARTESIAN_POINT ( 'NONE',  ( 27.24857305709999977, -7.138312704079999627, 229.9172022069999741 ) ) ;
#27924=CARTESIAN_POINT ( 'NONE',  ( -0.2818134472887923181, -12.32633712609394294, 232.6627637456880677 ) ) ;
#27946=VERTEX_POINT ( 'NONE', #18157 ) ;
#27950=CARTESIAN_POINT ( 'NONE',  ( -17.99591469510000152, 19.96082041680000074, 229.9999991770000065 ) ) ;
#27978=EDGE_LOOP ( 'NONE', ( #29830, #23675, #22532, #20349 ) ) ;
#28011=CARTESIAN_POINT ( 'NONE',  ( -24.60699806910000120, -12.93667933180000063, 224.8957833819999621 ) ) ;
#28017=VERTEX_POINT ( 'NONE', #30453 ) ;
#28018=CARTESIAN_POINT ( 'NONE',  ( 2.131628207279999844E-14, -1.704192342799999938E-14, 230.0904314459999966 ) ) ;
#28020=CARTESIAN_POINT ( 'NONE',  ( -22.83911234509999844, 16.42879871570000105, 229.0000000010000178 ) ) ;
#28037=CARTESIAN_POINT ( 'NONE',  ( -24.09883371379999772, -15.21565466309999870, 225.1042187089999800 ) ) ;
#28038=EDGE_CURVE ( 'NONE', #23898, #11807, #9466, .T. ) ;
#28051=CARTESIAN_POINT ( 'NONE',  ( -24.91946588839999777, -13.83134141909999926, 226.0028092389999870 ) ) ;
#28064=CARTESIAN_POINT ( 'NONE',  ( 24.91104292519999674, -14.27662681390000010, 229.9172020129999794 ) ) ;
#28066=CARTESIAN_POINT ( 'NONE',  ( 8.460443391580000139, -26.64180382800000046, 222.0000000000000000 ) ) ;
#28073=CARTESIAN_POINT ( 'NONE',  ( 6.422810853499230532, 10.52452000602716708, 232.6627635423665481 ) ) ;
#28097=CARTESIAN_POINT ( 'NONE',  ( -11.28020519024417823, 4.977446647725678019, 232.6627637660202765 ) ) ;
#28101=ADVANCED_FACE ( 'NONE', ( #19259 ), #9791, .F. ) ;
#28117=CARTESIAN_POINT ( 'NONE',  ( 24.64642659020000082, -14.31106159850000026, 226.0986569330000293 ) ) ;
#28118=CARTESIAN_POINT ( 'NONE',  ( 19.18299057799999829, 20.00000421109999849, 230.4461458050000147 ) ) ;
#28133=CARTESIAN_POINT ( 'NONE',  ( -24.48873108240000107, -14.58042505439999914, 223.9574921880000034 ) ) ;
#28145=CARTESIAN_POINT ( 'NONE',  ( -21.70990266010000269, 18.50700188859999784, 225.0000000000000000 ) ) ;
#28150=CARTESIAN_POINT ( 'NONE',  ( -13.25572673970000004, -26.61578565920000017, 230.6999999999999886 ) ) ;
#28152=CARTESIAN_POINT ( 'NONE',  ( 27.30137319059999967, 6.660265673030000499, 222.0000000000000000 ) ) ;
#28177=B_SPLINE_CURVE_WITH_KNOTS ( 'NONE', 5,
 ( #22868, #8841, #23026, #18126, #18446, #4132 ),
 .UNSPECIFIED., .F., .F.,
 ( 6, 6 ),
 ( -7.000000000120000010, -4.999999893120000038 ),
 .UNSPECIFIED. ) ;
#28178=CARTESIAN_POINT ( 'NONE',  ( -27.79999999980000069, 4.328052719890000510, 229.0000000000000000 ) ) ;
#28192=DIRECTION ( 'NONE',  ( -0.2665630446479613780, -0.9085064176298685013, -0.3218077568259533061 ) ) ;
#28193=CARTESIAN_POINT ( 'NONE',  ( -24.64674669160000064, -14.31123007319999907, 226.0986578890000089 ) ) ;
#28200=CARTESIAN_POINT ( 'NONE',  ( -21.99953312579999931, 17.62920693399999905, 229.1414213380000149 ) ) ;
#28201=ORIENTED_EDGE ( 'NONE', *, *, #5449, .F. ) ;
#28217=CARTESIAN_POINT ( 'NONE',  ( 5.229687933670000177, -30.84198039099999633, 228.9999999970000317 ) ) ;
#28220=CARTESIAN_POINT ( 'NONE',  ( 28.39965777970000005, -2.618405453069999833, 222.0000000000000000 ) ) ;
#28231=FACE_OUTER_BOUND ( 'NONE', #19084, .T. ) ;
#28237=ADVANCED_FACE ( 'NONE', ( #17804 ), #19339, .F. ) ;
#28239=CARTESIAN_POINT ( 'NONE',  ( 19.80538173169999894, 19.50875421069999760, 224.8000000000000114 ) ) ;
#28244=( LENGTH_UNIT ( ) NAMED_UNIT ( * ) SI_UNIT ( .MILLI., .METRE. ) );
#28247=CARTESIAN_POINT ( 'NONE',  ( -4.456723305595252427, 11.49589586079882686, 232.6627637660202765 ) ) ;
#28260=B_SPLINE_SURFACE_WITH_KNOTS ( 'NONE', 5, 5, ( 
 ( #17340, #10111, #19709, #15588, #17634, #29292, #27243, #10266, #29755 ),
 ( #27550, #8186, #5683, #17785, #25042, #26944, #19869, #5530, #3473 ),
 ( #29450, #22680, #1125, #5993, #10716, #17489, #5380, #20313, #29915 ),
 ( #8340, #14987, #25194, #3627, #22221, #24584, #3018, #12611, #16066 ),
 ( #1906, #6313, #18255, #23471, #13865, #23308, #3951, #27864, #30224 ),
 ( #15746, #22835, #6776, #25357, #23157, #15908, #8977, #25674, #25516 ) ),
 .UNSPECIFIED., .F., .F., .F.,
 ( 6, 6 ),
 ( 6, 3, 6 ),
 ( 0.000000000000000000, 23.80447727570000183 ),
 ( 8.011061266649999624, 9.372204729519999944, 10.73334819239999938 ),
 .UNSPECIFIED. ) ;
#28278=CARTESIAN_POINT ( 'NONE',  ( -20.30396346383280104, 20.00000000000023803, 229.1317800523452775 ) ) ;
#28282=CARTESIAN_POINT ( 'NONE',  ( -23.83777999500000178, -14.30502388280000048, 223.9971937000000253 ) ) ;
#28301=CARTESIAN_POINT ( 'NONE',  ( 5.185037338370000803, -30.57858919520000285, 230.5592437530000041 ) ) ;
#28302=ORIENTED_EDGE ( 'NONE', *, *, #9715, .F. ) ;
#28308=CARTESIAN_POINT ( 'NONE',  ( 0.4702670923129999569, -27.79645255899999867, 223.9974824469999817 ) ) ;
#28315=AXIS2_PLACEMENT_3D ( 'NONE', #9468, #7111, #16695 ) ;
#28320=CARTESIAN_POINT ( 'NONE',  ( -24.68204616399999907, -14.25020164319999871, 223.9000014189999774 ) ) ;
#28325=ORIENTED_EDGE ( 'NONE', *, *, #20743, .T. ) ;
#28330=VERTEX_POINT ( 'NONE', #26303 ) ;
#28331=CARTESIAN_POINT ( 'NONE',  ( -25.11765555659999904, -13.46780168200000105, 225.6808342349999918 ) ) ;
#28339=CARTESIAN_POINT ( 'NONE',  ( -19.80526744909999692, 19.50877353739999975, 229.0000000010000178 ) ) ;
#28351=CARTESIAN_POINT ( 'NONE',  ( -24.11911872370000154, -15.18353100999999938, 225.3106464589999973 ) ) ;
#28355=ORIENTED_EDGE ( 'NONE', *, *, #1132, .T. ) ;
#28358=CARTESIAN_POINT ( 'NONE',  ( -24.76252940850000073, 13.73644554549999874, 229.4485733019999998 ) ) ;
#28363=CARTESIAN_POINT ( 'NONE',  ( 19.80538173680000114, 19.50875419940000199, 226.9999998930000231 ) ) ;
#28380=CARTESIAN_POINT ( 'NONE',  ( 20.00949237780000090, -20.13757562109999810, 230.0000000000000000 ) ) ;
#28385=CARTESIAN_POINT ( 'NONE',  ( 0.4821455018050000429, -28.49635764770000179, 226.0025203910000187 ) ) ;
#28390=AXIS2_PLACEMENT_3D ( 'NONE', #11454, #30337, #11607 ) ;
#28391=CARTESIAN_POINT ( 'NONE',  ( 11.28020549271892570, -4.977446785437388499, 232.6627636541932702 ) ) ;
#28396=CARTESIAN_POINT ( 'NONE',  ( -27.79999999169999825, 0.8519339693649999878, 222.0000000000000000 ) ) ;
#28416=CARTESIAN_POINT ( 'NONE',  ( -19.80526744929999694, 19.50877353739999975, 229.0739196179999908 ) ) ;
#28427=CARTESIAN_POINT ( 'NONE',  ( 24.62873585949999722, -14.34148440729999940, 226.0959678990000157 ) ) ;
#28430=CARTESIAN_POINT ( 'NONE',  ( -25.27355175290000133, 12.75978488059999805, 229.0000000000000000 ) ) ;
#28433=B_SPLINE_CURVE_WITH_KNOTS ( 'NONE', 5,
 ( #22206, #25179, #20454, #6132, #1270, #27079, #10870, #30051, #15725, #5517, #15120, #24718, #12754, #22366, #10401 ),
 .UNSPECIFIED., .F., .F.,
 ( 6, 3, 3, 3, 6 ),
 ( 0.000000000000000000, 0.09999999999828219910, 0.3999999999988547716, 0.6999999999999999556, 1.000000000000000000 ),
 .UNSPECIFIED. ) ;
#28443=CARTESIAN_POINT ( 'NONE',  ( -24.04140365350000152, -13.95971772459999904, 223.9013449489999914 ) ) ;
#28459=CARTESIAN_POINT ( 'NONE',  ( -14.07565872370000015, -28.26210308950000183, 229.4982322489999831 ) ) ;
#28461=CARTESIAN_POINT ( 'NONE',  ( -24.64674669169999888, -14.31123007319999907, 223.9013449489999914 ) ) ;
#28466=CARTESIAN_POINT ( 'NONE',  ( 1.089891362619999970, -28.47934442809999922, 224.6898179359999972 ) ) ;
#28483=EDGE_CURVE ( 'NONE', #55, #15092, #16205, .T. ) ;
#28497=CARTESIAN_POINT ( 'NONE',  ( -18.03086237940000203, 20.00000062619999852, 230.7000111870000012 ) ) ;
#28508=CARTESIAN_POINT ( 'NONE',  ( 27.79999999999999716, 2.355323124549999985E-11, 229.1414213560000235 ) ) ;
#28513=CARTESIAN_POINT ( 'NONE',  ( -17.83931601680000156, 20.00000000000000000, 230.0000000000000000 ) ) ;
#28535=CARTESIAN_POINT ( 'NONE',  ( -21.68201525099999927, -17.64200409929999935, 222.0000000000000000 ) ) ;
#28536=CARTESIAN_POINT ( 'NONE',  ( 0.3832430167449999980, -28.49789927060000139, 226.0423291289999952 ) ) ;
#28542=CARTESIAN_POINT ( 'NONE',  ( 7.265485053589353370, -9.961462563069886755, 232.6627636948576878 ) ) ;
#28557=CARTESIAN_POINT ( 'NONE',  ( 28.50000000000000000, 1.065814103639999922E-14, 229.0000000000000000 ) ) ;
#28586=CARTESIAN_POINT ( 'NONE',  ( 19.36601073090000114, 20.00000521309999968, 230.3593855350000013 ) ) ;
#28587=FACE_OUTER_BOUND ( 'NONE', #21932, .T. ) ;
#28589=CARTESIAN_POINT ( 'NONE',  ( -0.6685465368700000965, -28.49273882800000024, 225.9009104920000084 ) ) ;
#28602=CARTESIAN_POINT ( 'NONE',  ( -23.88727024800000009, -14.22229899360000083, 223.9574921880000034 ) ) ;
#28614=CARTESIAN_POINT ( 'NONE',  ( -22.97691952320000297, 16.89267704250000079, 223.0000000000000000 ) ) ;
#28618=CARTESIAN_POINT ( 'NONE',  ( -23.31151963009999761, -20.60626745989999975, 230.2432540810000319 ) ) ;
#28642=VERTEX_POINT ( 'NONE', #5893 ) ;
#28643=CARTESIAN_POINT ( 'NONE',  ( -0.6521609807820000215, -27.79292263629999837, 224.0990923460000204 ) ) ;
#28689=CARTESIAN_POINT ( 'NONE',  ( 0.1059454459490000028, -28.50005195860000029, 226.0959520840000039 ) ) ;
#28728=CARTESIAN_POINT ( 'NONE',  ( -5.304254813150000639E-10, 4.380584783799999468E-10, 230.0000000000000000 ) ) ;
#28729=CARTESIAN_POINT ( 'NONE',  ( 24.55806919409999978, -14.46257963250000067, 226.0798541909999813 ) ) ;
#28730=CARTESIAN_POINT ( 'NONE',  ( -10.18299983019999821, -6.475798291150000274, 231.9999989789999972 ) ) ;
#28734=CARTESIAN_POINT ( 'NONE',  ( -0.8738876050170000243, -27.78662806160000187, 225.6801695290000112 ) ) ;
#28745=CONICAL_SURFACE ( 'NONE', #22223, 11.99999999999999467, 1.243158134259999770 ) ;
#28749=VERTEX_POINT ( 'NONE', #23689 ) ;
#28761=CARTESIAN_POINT ( 'NONE',  ( -22.91194469939999934, -20.25306243529999861, 230.5592437530000041 ) ) ;
#28763=CARTESIAN_POINT ( 'NONE',  ( -24.25909092259999866, -14.95913241689999928, 224.2397348780000073 ) ) ;
#28765=CARTESIAN_POINT ( 'NONE',  ( -27.79999999999999716, -2.359477751120000078E-11, 227.5999999999999943 ) ) ;
#28768=CARTESIAN_POINT ( 'NONE',  ( 19.80538173169999894, 19.50875421069999760, 226.9999998930000231 ) ) ;
#28778=CARTESIAN_POINT ( 'NONE',  ( 7.768677137030000068, 16.06355773770000184, 230.7531949689999919 ) ) ;
#28779=ORIENTED_EDGE ( 'NONE', *, *, #22083, .T. ) ;
#28786=CARTESIAN_POINT ( 'NONE',  ( -0.1033151399490000039, -27.80006701330000141, 223.9040511909999793 ) ) ;
#28787=ORIENTED_EDGE ( 'NONE', *, *, #2788, .F. ) ;
#28795=CARTESIAN_POINT ( 'NONE',  ( -19.76603762889999771, 19.51852293520000003, 229.2245375310000099 ) ) ;
#28806=B_SPLINE_CURVE_WITH_KNOTS ( 'NONE', 5,
 ( #4589, #4290, #16235, #25851, #9467, #14045, #21274, #28508, #23496 ),
 .UNSPECIFIED., .F., .F.,
 ( 6, 3, 6 ),
 ( 8.011061266649999624, 8.831591450809998634, 9.652121634960000307 ),
 .UNSPECIFIED. ) ;
#28815=CARTESIAN_POINT ( 'NONE',  ( 24.80399018339999628, -14.03663607480000053, 226.0798554400000171 ) ) ;
#28844=CARTESIAN_POINT ( 'NONE',  ( 28.49999999990000177, 2.434992796449999553, 222.0000000000000000 ) ) ;
#28853=CARTESIAN_POINT ( 'NONE',  ( 28.50000000000000000, 8.881784197000000993E-16, 222.0000000000000000 ) ) ;
#28854=CARTESIAN_POINT ( 'NONE',  ( 17.83931934270000141, 20.00000000000000000, 230.3499999999999943 ) ) ;
#28873=CARTESIAN_POINT ( 'NONE',  ( 2.131628207279999844E-14, 1.421085471519999843E-14, 230.0904314459999966 ) ) ;
#28881=CARTESIAN_POINT ( 'NONE',  ( 23.56533302370000271, -14.74861233630000079, 224.4930104139999969 ) ) ;
#28894=ADVANCED_FACE ( 'NONE', ( #16732 ), #19595, .T. ) ;
#28900=CARTESIAN_POINT ( 'NONE',  ( 9.777910293735976310, 7.131609509313695305, 232.0000002394077683 ) ) ;
#28906=CARTESIAN_POINT ( 'NONE',  ( -24.12724309970000292, -13.81083407110000039, 223.9040321390000088 ) ) ;
#28908=CARTESIAN_POINT ( 'NONE',  ( 24.53709010086652142, -14.49830767851621793, 223.9262482216262242 ) ) ;
#28921=CARTESIAN_POINT ( 'NONE',  ( 3.974243191089999350, 11.57455430929999984, 232.6627648150000027 ) ) ;
#28936=EDGE_CURVE ( 'NONE', #1204, #5832, #27779, .T. ) ;
#28939=EDGE_CURVE ( 'NONE', #979, #13384, #6046, .T. ) ;
#28952=CARTESIAN_POINT ( 'NONE',  ( -0.4820778521899999891, -28.49640832880000119, 223.9974845609999932 ) ) ;
#28962=EDGE_CURVE ( 'NONE', #29947, #17135, #18422, .T. ) ;
#28974=CARTESIAN_POINT ( 'NONE',  ( 24.07552309629999954, -13.90001137839999856, 223.9000014189999774 ) ) ;
#28981=CARTESIAN_POINT ( 'NONE',  ( 24.69936741169999905, -14.21947533890000059, 226.1000014189999945 ) ) ;
#28988=CARTESIAN_POINT ( 'NONE',  ( -21.16705332929999983, 21.30254446269999846, 222.0000000000000000 ) ) ;
#29001=CARTESIAN_POINT ( 'NONE',  ( 28.50000000000000000, 8.881784197000000993E-16, 222.0000000000000000 ) ) ;
#29005=CARTESIAN_POINT ( 'NONE',  ( 24.61862080450000079, 14.40921680009999939, 222.0000000000000000 ) ) ;
#29009=CARTESIAN_POINT ( 'NONE',  ( 21.55746468670000127, 17.28477200280000048, 229.9172016159999998 ) ) ;
#29010=CARTESIAN_POINT ( 'NONE',  ( -18.35450744919999977, 0.3144422474040000082, 230.6999999999999886 ) ) ;
#29024=ORIENTED_EDGE ( 'NONE', *, *, #70, .F. ) ;
#29040=CARTESIAN_POINT ( 'NONE',  ( -6.530148857409999508, -10.14823162649999944, 231.9999989789999972 ) ) ;
#29042=CARTESIAN_POINT ( 'NONE',  ( -12.09920997781542873, 0.2766207017873786866, 232.0000000000048033 ) ) ;
#29058=ADVANCED_FACE ( 'NONE', ( #16396 ), #21790, .T. ) ;
#29060=CARTESIAN_POINT ( 'NONE',  ( 24.80399018339999628, -14.03663607480000053, 226.0798554400000171 ) ) ;
#29068=ORIENTED_EDGE ( 'NONE', *, *, #18911, .T. ) ;
#29086=B_SPLINE_CURVE_WITH_KNOTS ( 'NONE', 5,
 ( #24484, #15185, #27299, #26995, #29188, #9852, #5434, #17684, #24943, #5585, #7489, #29504, #19918, #27150, #24635 ),
 .UNSPECIFIED., .F., .F.,
 ( 6, 3, 3, 3, 6 ),
 ( 0.000000000000000000, 0.1000000000011452422, 0.4000000000045809689, 0.7000000000005726086, 1.000000000000000000 ),
 .UNSPECIFIED. ) ;
#29090=CARTESIAN_POINT ( 'NONE',  ( -21.99953312590000110, 17.62920693369999725, 229.0000000010000178 ) ) ;
#29102=CARTESIAN_POINT ( 'NONE',  ( -0.8057362888000000334, -27.78873281839999976, 224.2403608809999866 ) ) ;
#29111=CARTESIAN_POINT ( 'NONE',  ( -22.41257468390000085, 16.47776880720000037, 223.0000000000000000 ) ) ;
#29113=CARTESIAN_POINT ( 'NONE',  ( -133283.2115610000037, -454258.9661130000022, -160669.8390839999774 ) ) ;
#29155=CARTESIAN_POINT ( 'NONE',  ( 24.01396915060000126, 14.05529641579999911, 222.0000000000000000 ) ) ;
#29161=ORIENTED_EDGE ( 'NONE', *, *, #8815, .F. ) ;
#29186=CARTESIAN_POINT ( 'NONE',  ( -10.27234744519999943, 6.417650034250000246, 231.9999989789999972 ) ) ;
#29188=CARTESIAN_POINT ( 'NONE',  ( 23.95489023949999918, -14.10735628980000023, 223.9201486480000085 ) ) ;
#29203=DIRECTION ( 'NONE',  ( 1.000000000000000000, 0.000000000000000000, 0.000000000000000000 ) ) ;
#29215=CARTESIAN_POINT ( 'NONE',  ( -25.17013648539154147, -13.36928061894358244, 224.5014256759218370 ) ) ;
#29217=B_SPLINE_SURFACE_WITH_KNOTS ( 'NONE', 5, 1, ( 
 ( #13805, #30952 ),
 ( #18983, #23252 ),
 ( #25772, #2321 ),
 ( #1849, #11903 ),
 ( #6559, #16772 ),
 ( #9224, #28734 ),
 ( #30495, #25927 ),
 ( #28589, #4362 ),
 ( #13648, #13965 ),
 ( #16467, #23576 ),
 ( #26081, #4520 ),
 ( #31105, #14118 ),
 ( #7031, #23722 ),
 ( #2161, #11749 ),
 ( #16620, #26228 ) ),
 .UNSPECIFIED., .F., .F., .F.,
 ( 6, 3, 3, 3, 6 ),
 ( 2, 2 ),
 ( 0.000000000000000000, 0.5239015562240000312, 1.047803112450000018, 1.571704668670000027, 1.746338520749999956 ),
 ( -0.7000000000009999335, 2.556819966299999618E-06 ),
 .UNSPECIFIED. ) ;
#29219=CARTESIAN_POINT ( 'NONE',  ( 6.460394865750000548, 10.46154704049999928, 232.6627648150000027 ) ) ;
#29224=EDGE_LOOP ( 'NONE', ( #6540, #12269, #9059, #5715 ) ) ;
#29238=CARTESIAN_POINT ( 'NONE',  ( -26.73216212440000206, 9.347130611989999949, 229.4485730460000070 ) ) ;
#29252=CARTESIAN_POINT ( 'NONE',  ( 20.11799773827349824, 19.99998646409962433, 229.6587445809824146 ) ) ;
#29263=CARTESIAN_POINT ( 'NONE',  ( -23.79652740965775237, -14.37370918960761657, 224.0358530723576393 ) ) ;
#29270=CARTESIAN_POINT ( 'NONE',  ( -28.50000000000000000, -5.684341886079999373E-14, 229.0000000000000000 ) ) ;
#29271=CARTESIAN_POINT ( 'NONE',  ( 0.9902601296000002051, -27.78262976010000074, 225.5064715119999903 ) ) ;
#29292=CARTESIAN_POINT ( 'NONE',  ( 28.35924375250000296, 3.617365304089999312E-14, 229.7625741969999922 ) ) ;
#29306=CARTESIAN_POINT ( 'NONE',  ( 27.79999999460000026, 2.375185947459999891, 222.0000000000000000 ) ) ;
#29309=CARTESIAN_POINT ( 'NONE',  ( 26.12735226819999923, 9.150265136599999849, 229.9751247030000059 ) ) ;
#29354=FILL_AREA_STYLE ('',( #5590 ) ) ;
#29359=ORIENTED_EDGE ( 'NONE', *, *, #7674, .T. ) ;
#29361=CARTESIAN_POINT ( 'NONE',  ( 24.71695093370000151, -14.18891100779999981, 226.0986570600000221 ) ) ;
#29372=CARTESIAN_POINT ( 'NONE',  ( 0.000000000000000000, 0.000000000000000000, 230.0000000000000000 ) ) ;
#29376=CARTESIAN_POINT ( 'NONE',  ( 11.47889647200000063, 4.402643528619999636, 232.6627648150000027 ) ) ;
#29381=CARTESIAN_POINT ( 'NONE',  ( 28.04325408110000240, -4.263256414559999688E-14, 230.2432540810000319 ) ) ;
#29388=DIRECTION ( 'NONE',  ( 0.000000000000000000, 0.000000000000000000, 1.000000000000000000 ) ) ;
#29390=AXIS2_PLACEMENT_3D ( 'NONE', #1692, #3568, #25457 ) ;
#29391=CARTESIAN_POINT ( 'NONE',  ( -23.50695067596906185, -14.84192170558064738, 225.0734924212516432 ) ) ;
#29395=CARTESIAN_POINT ( 'NONE',  ( -19.41377926560965506, 19.99999670840111676, 230.3187478872601162 ) ) ;
#29396=CARTESIAN_POINT ( 'NONE',  ( -27.09307779339999911, -1.459449460099999974E-12, 229.9751247039999953 ) ) ;
#29420=VERTEX_POINT ( 'NONE', #4403 ) ;
#29424=CARTESIAN_POINT ( 'NONE',  ( 0.9559440766510057808, -27.78378678420316206, 225.5621479832471437 ) ) ;
#29427=CARTESIAN_POINT ( 'NONE',  ( -24.47688144805034938, -13.18130191084491010, 225.7329853482806357 ) ) ;
#29443=VERTEX_POINT ( 'NONE', #2205 ) ;
#29450=CARTESIAN_POINT ( 'NONE',  ( 25.84472112319999937, 9.051226241569999331, 230.6999999999999886 ) ) ;
#29451=CARTESIAN_POINT ( 'NONE',  ( -28.49999999979999998, 7.466149641079999455, 222.0000000000000000 ) ) ;
#29454=CARTESIAN_POINT ( 'NONE',  ( -20.30396346370000060, 20.00000000000000000, 228.1999999999999886 ) ) ;
#29459=B_SPLINE_CURVE_WITH_KNOTS ( 'NONE', 5,
 ( #10808, #20402, #755, #10346, #29989, #15671, #25283, #3718, #19939 ),
 .UNSPECIFIED., .F., .F.,
 ( 6, 3, 6 ),
 ( 0.000000000000000000, 54.03331039209999886, 92.56095350929999199 ),
 .UNSPECIFIED. ) ;
#29481=VERTEX_POINT ( 'NONE', #2511 ) ;
#29484=VERTEX_POINT ( 'NONE', #11943 ) ;
#29486=CARTESIAN_POINT ( 'NONE',  ( -23.08867861179999892, -20.40921893140000165, 229.2930746810000073 ) ) ;
#29498=CARTESIAN_POINT ( 'NONE',  ( 18.92330595649999836, 19.72869720889999812, 229.8506619570000282 ) ) ;
#29504=CARTESIAN_POINT ( 'NONE',  ( 23.52644129050000288, -14.81042608839999808, 224.6894478949999723 ) ) ;
#29529=CARTESIAN_POINT ( 'NONE',  ( -25.09216856445464927, -13.51511586023699785, 224.2647128708496211 ) ) ;
#29544=CARTESIAN_POINT ( 'NONE',  ( 24.07552309629999954, -13.90001137829999855, 226.1000014189999945 ) ) ;
#29545=CARTESIAN_POINT ( 'NONE',  ( -23.62704991831892798, -14.65035393207314840, 225.6826156241376111 ) ) ;
#29550=CARTESIAN_POINT ( 'NONE',  ( -18.06506883821712961, 19.99992188150034877, 230.6935433854662847 ) ) ;
#29575=CARTESIAN_POINT ( 'NONE',  ( -24.00379068851701447, -14.02496465848369844, 223.9000014189999774 ) ) ;
#29583=CARTESIAN_POINT ( 'NONE',  ( -24.34628147195961390, -13.42155311436081355, 225.9641454712443078 ) ) ;
#29585=CARTESIAN_POINT ( 'NONE',  ( 0.6521647005340001080, -27.79285400239999859, 225.9009072510000067 ) ) ;
#29670=CARTESIAN_POINT ( 'NONE',  ( 14.09657531829999932, 28.30410039250000054, 229.0000000000000000 ) ) ;
#29716=VERTEX_POINT ( 'NONE', #22945 ) ;
#29748=CARTESIAN_POINT ( 'NONE',  ( -19.80526744909999692, 19.50877353739999975, 229.0000000010000178 ) ) ;
#29752=ORIENTED_EDGE ( 'NONE', *, *, #12946, .F. ) ;
#29755=CARTESIAN_POINT ( 'NONE',  ( 28.50000000000000000, 3.197442310919999608E-14, 229.0000000000000000 ) ) ;
#29764=EDGE_CURVE ( 'NONE', #18684, #7240, #18370, .T. ) ;
#29771=CARTESIAN_POINT ( 'NONE',  ( -17.99934820270000202, 20.17941515389999907, 230.6999999999999886 ) ) ;
#29773=EDGE_CURVE ( 'NONE', #18419, #29716, #11235, .T. ) ;
#29774=CARTESIAN_POINT ( 'NONE',  ( -13.75032424529999986, -27.60893268180000248, 229.0000000000000000 ) ) ;
#29775=CARTESIAN_POINT ( 'NONE',  ( 9.987902756569999596, 15.20391984080000114, 230.6999999999999886 ) ) ;
#29794=CARTESIAN_POINT ( 'NONE',  ( -26.94142135619999934, -9.898318926829999143, 230.0000000000000000 ) ) ;
#29796=CARTESIAN_POINT ( 'NONE',  ( -27.72015578919999967, -7.265888686289999399, 222.0000000000000000 ) ) ;
#29805=CARTESIAN_POINT ( 'NONE',  ( 25.17364887440000132, -13.36205984489999921, 224.4930265309999982 ) ) ;
#29816=CARTESIAN_POINT ( 'NONE',  ( -21.16705332919999805, 21.30254446269999846, 229.0000000000000000 ) ) ;
#29828=CARTESIAN_POINT ( 'NONE',  ( 18.31380613830149073, 20.00001766699981331, 230.6700634801132992 ) ) ;
#29830=ORIENTED_EDGE ( 'NONE', *, *, #17231, .T. ) ;
#29851=CARTESIAN_POINT ( 'NONE',  ( -23.53828869184600592, -14.79220260103408968, 225.3595846784022569 ) ) ;
#29856=CARTESIAN_POINT ( 'NONE',  ( -18.19349109261828090, 19.99999252024461072, 230.6834197065497563 ) ) ;
#29891=EDGE_CURVE ( 'NONE', #662, #18191, #11627, .T. ) ;
#29900=CONICAL_SURFACE ( 'NONE', #19853, 12.22526471199999598, 1.243158134259999770 ) ;
#29908=CARTESIAN_POINT ( 'NONE',  ( -24.39524108170000360, -13.33235248870000156, 224.0985996330000205 ) ) ;
#29915=CARTESIAN_POINT ( 'NONE',  ( 27.48412515190000249, 9.625371191550000205, 229.0000000000000000 ) ) ;
#29919=CARTESIAN_POINT ( 'NONE',  ( 5.361384718770000113, -31.61859215249999977, 222.0000000000000000 ) ) ;
#29929=CARTESIAN_POINT ( 'NONE',  ( -3.441895295100000141, -11.73074823080000151, 232.6627637660000119 ) ) ;
#29934=CARTESIAN_POINT ( 'NONE',  ( 18.35450725729999988, -0.3144534986609999749, 230.6999999999999886 ) ) ;
#29947=VERTEX_POINT ( 'NONE', #18990 ) ;
#29954=CARTESIAN_POINT ( 'NONE',  ( -27.79999999999999716, 2.356159711779999785E-11, 229.0000000000000000 ) ) ;
#29961=DIRECTION ( 'NONE',  ( 0.4353787270609800752, 0.9002473904559571416, 0.000000000000000000 ) ) ;
#29975=CARTESIAN_POINT ( 'NONE',  ( 25.26809621129999783, 12.77001316559999999, 226.2000000000000171 ) ) ;
#29989=CARTESIAN_POINT ( 'NONE',  ( 5.361384718760000112, -31.61859215249999977, 229.0000000000000000 ) ) ;
#29993=CARTESIAN_POINT ( 'NONE',  ( 1.127732790480000080, -28.47784299079999926, 225.0000014190000002 ) ) ;
#29994=EDGE_LOOP ( 'NONE', ( #7785, #25117, #23662, #24812 ) ) ;
#29997=CARTESIAN_POINT ( 'NONE',  ( 28.35924375250000296, -2.370246001849999498E-14, 229.7625741969999922 ) ) ;
#30006=CARTESIAN_POINT ( 'NONE',  ( 0.9837925379835922302, -27.78276979301110572, 224.5041803965649763 ) ) ;
#30011=CARTESIAN_POINT ( 'NONE',  ( -18.32656039618751009, 20.00000276249100395, 230.6693274794374986 ) ) ;
#30030=EDGE_CURVE ( 'NONE', #21281, #4391, #13858, .T. ) ;
#30033=CARTESIAN_POINT ( 'NONE',  ( 27.79999999980000069, -7.282770092339999835, 222.0000000000000000 ) ) ;
#30034=CARTESIAN_POINT ( 'NONE',  ( 24.09856112909999837, -15.21545593799999985, 225.0000014190000002 ) ) ;
#30046=CARTESIAN_POINT ( 'NONE',  ( 0.03443198226909999909, -27.80021999669999744, 226.1000014189999945 ) ) ;
#30049=CARTESIAN_POINT ( 'NONE',  ( 19.80538173989999962, 19.50875420239999869, 228.5999999789999890 ) ) ;
#30051=CARTESIAN_POINT ( 'NONE',  ( 0.6686231747119999458, -28.49266848160000265, 224.0990955869999937 ) ) ;
#30053=B_SPLINE_CURVE_WITH_KNOTS ( 'NONE', 1,
 ( #14314, #27715 ),
 .UNSPECIFIED., .F., .F.,
 ( 2, 2 ),
 ( -2.556023926959999973E-06, 0.7000000000009999335 ),
 .UNSPECIFIED. ) ;
#30061=CARTESIAN_POINT ( 'NONE',  ( -24.60699806910000120, -12.93667933180000063, 225.0000014190000002 ) ) ;
#30076=CARTESIAN_POINT ( 'NONE',  ( 21.16705260770000052, -21.30254494060000070, 222.0000000000000000 ) ) ;
#30089=CARTESIAN_POINT ( 'NONE',  ( -21.39843895140000285, 17.14751838560000152, 230.6999999999999886 ) ) ;
#30093=CARTESIAN_POINT ( 'NONE',  ( 5.229687933670000177, -30.84198039099999633, 229.0000000000000000 ) ) ;
#30094=CARTESIAN_POINT ( 'NONE',  ( -19.60939915890000051, -18.53226158640000065, 230.6999999999999886 ) ) ;
#30119=CARTESIAN_POINT ( 'NONE',  ( 6.830207510690000570E-10, 8.201972434560000246E-11, 230.0000000000000000 ) ) ;
#30125=CARTESIAN_POINT ( 'NONE',  ( 19.56378028550000181, 19.56885116670000357, 229.4995147189999898 ) ) ;
#30136=CARTESIAN_POINT ( 'NONE',  ( 26.95545381250000361, 8.667969360479998997, 223.3999999999999773 ) ) ;
#30144=CARTESIAN_POINT ( 'NONE',  ( 24.07552037900000030, -13.90000980950000020, 226.1000014189999945 ) ) ;
#30150=ORIENTED_EDGE ( 'NONE', *, *, #20847, .F. ) ;
#30157=CARTESIAN_POINT ( 'NONE',  ( -0.06887222117169999880, -27.80017212539999960, 223.9013489249999793 ) ) ;
#30161=CARTESIAN_POINT ( 'NONE',  ( 1.099998580829999906, -27.77839262550000043, 225.0000014190000002 ) ) ;
#30173=CARTESIAN_POINT ( 'NONE',  ( -20.21685729201897175, 19.99998469724611283, 229.4596784481962288 ) ) ;
#30197=CARTESIAN_POINT ( 'NONE',  ( 27.79999999999999716, -2.355626804729999831E-11, 222.0000000000000000 ) ) ;
#30223=EDGE_LOOP ( 'NONE', ( #16748, #24145, #18849 ) ) ;
#30224=CARTESIAN_POINT ( 'NONE',  ( 22.54750148980000191, 18.07861229629999755, 229.0000000000000000 ) ) ;
#30229=CARTESIAN_POINT ( 'NONE',  ( -28.49999999970000175, -10.47094308429999998, 222.0000000000000000 ) ) ;
#30234=CARTESIAN_POINT ( 'NONE',  ( -1.015151870880000029, -28.48229306780000059, 225.5064930660000186 ) ) ;
#30244=CARTESIAN_POINT ( 'NONE',  ( -28.50000000000000000, -5.504861435589999933E-14, 229.0000000000000000 ) ) ;
#30249=CARTESIAN_POINT ( 'NONE',  ( -27.79999999999999716, 2.355804440410000085E-11, 229.0000000000000000 ) ) ;
#30250=CARTESIAN_POINT ( 'NONE',  ( 17.91346439750000386, -3.648009858620000045, 230.6999999999999886 ) ) ;
#30265=EDGE_LOOP ( 'NONE', ( #14921, #8501, #28355, #22102 ) ) ;
#30273=CARTESIAN_POINT ( 'NONE',  ( 26.80000000000000071, -5.684341886079999373E-14, 230.0000000000000000 ) ) ;
#30275=CARTESIAN_POINT ( 'NONE',  ( -27.79999999999999716, 2.355410854109999913E-11, 222.0000000000000000 ) ) ;
#30284=ORIENTED_EDGE ( 'NONE', *, *, #19819, .F. ) ;
#30285=CARTESIAN_POINT ( 'NONE',  ( 25.08428924680000094, -13.52916357279999993, 224.2398747240000034 ) ) ;
#30287=CARTESIAN_POINT ( 'NONE',  ( -27.79999999180000358, -2.354738626309999853E-11, 222.0000000000000000 ) ) ;
#30297=CARTESIAN_POINT ( 'NONE',  ( 25.26809617030000155, 12.77001320659999983, 227.5999999999999943 ) ) ;
#30302=( NAMED_UNIT ( * ) SI_UNIT ( $, .STERADIAN. ) SOLID_ANGLE_UNIT ( ) );
#30308=CARTESIAN_POINT ( 'NONE',  ( 20.14371221788036692, 19.99999315982380210, 229.6128283330888848 ) ) ;
#30311=CARTESIAN_POINT ( 'NONE',  ( -19.80526744909999692, 19.50877353739999975, 229.0000000010000178 ) ) ;
#30329=CARTESIAN_POINT ( 'NONE',  ( -24.22223838309999877, -15.01863363589999878, 225.6808321819999890 ) ) ;
#30337=DIRECTION ( 'NONE',  ( 0.9595496299847263710, -0.2815395311429191305, 0.000000000000000000 ) ) ;
#30358=CARTESIAN_POINT ( 'NONE',  ( -5.112571995710000650, -10.85828497149999983, 231.9999991140000191 ) ) ;
#30362=FACE_OUTER_BOUND ( 'NONE', #20264, .T. ) ;
#30370=CARTESIAN_POINT ( 'NONE',  ( 0.07063658732710000054, -28.50016343120000073, 223.9013487590000011 ) ) ;
#30398=CARTESIAN_POINT ( 'NONE',  ( -24.60699806910000120, -12.93667933180000063, 225.0000014190000002 ) ) ;
#30417=CARTESIAN_POINT ( 'NONE',  ( 20.64716981389999972, -20.77933506589999979, 229.0000000000000000 ) ) ;
#30441=CARTESIAN_POINT ( 'NONE',  ( 24.50094951250000008, -14.04160150939999951, 230.0000000000000000 ) ) ;
#30443=CARTESIAN_POINT ( 'NONE',  ( 19.20441074659999714, -21.26949966540000148, 222.0000000000000000 ) ) ;
#30453=CARTESIAN_POINT ( 'NONE',  ( -1.127665019380000189, -28.47796022459999676, 225.0000014190000002 ) ) ;
#30454=CARTESIAN_POINT ( 'NONE',  ( 28.50000000000000000, -1.056438886989999914E-13, 222.0000000000000000 ) ) ;
#30495=CARTESIAN_POINT ( 'NONE',  ( -0.8259893078309999970, -28.48844349870000059, 225.7596419580000315 ) ) ;
#30500=CARTESIAN_POINT ( 'NONE',  ( -20.19118766868406212, 19.99999867976873702, 229.5201436231253354 ) ) ;
#30516=CARTESIAN_POINT ( 'NONE',  ( -23.55406855550000245, 16.04544956020000157, 222.0000000000000000 ) ) ;
#30518=CARTESIAN_POINT ( 'NONE',  ( -23.55406855550000245, 16.04544956020000157, 222.0000000000000000 ) ) ;
#30522=CARTESIAN_POINT ( 'NONE',  ( -23.57419247189999822, -20.83845762109999811, 229.7625741969999922 ) ) ;
#30531=B_SPLINE_SURFACE_WITH_KNOTS ( 'NONE', 5, 5, ( 
 ( #6033, #19904, #3672, #20361, #20202, #27135, #22575, #8544, #29954 ),
 ( #3840, #29794, #27437, #25407, #8382, #5569, #8226, #5873, #13272 ),
 ( #15483, #15170, #10308, #23046, #13428, #22885, #29486, #1327, #18144 ),
 ( #17528, #6194, #15795, #7925, #24775, #12818, #22422, #11231, #6508 ),
 ( #23362, #1642, #16108, #6820, #18930, #18619, #20836, #1490, #28217 ),
 ( #16569, #28380, #20677, #21145, #9170, #23199, #16416, #25877, #18772 ),
 ( #30441, #11698, #25720, #28064, #2104, #23670, #1952, #13748, #4153 ),
 ( #14218, #25560, #11081, #27914, #8861, #1801, #8701, #21299, #9021 ),
 ( #30273, #18309, #3997, #30901, #30740, #26175, #15952, #13908, #13594 ) ),
 .UNSPECIFIED., .F., .F., .F.,
 ( 6, 3, 6 ),
 ( 6, 3, 6 ),
 ( 0.000000000000000000, 53.20205529499999386, 91.13698440880000362 ),
 ( 8.011061266649999624, 8.831591450809998634, 9.652121634960000307 ),
 .UNSPECIFIED. ) ;
#30559=CARTESIAN_POINT ( 'NONE',  ( -19.90459424020000156, 20.00000653480000068, 229.9504594400000030 ) ) ;
#30569=CARTESIAN_POINT ( 'NONE',  ( -23.52673845780000050, -14.81058795080000046, 225.3106464589999973 ) ) ;
#30593=CARTESIAN_POINT ( 'NONE',  ( 28.50000000000000000, 1.065814103639999922E-14, 229.0000000000000000 ) ) ;
#30597=CARTESIAN_POINT ( 'NONE',  ( -12.43585889439999903, -25.03430743100000200, 222.0000000000000000 ) ) ;
#30602=EDGE_CURVE ( 'NONE', #18191, #30960, #25548, .T. ) ;
#30604=CARTESIAN_POINT ( 'NONE',  ( 5.114250173089999407, 17.43050732989999929, 230.0000000000000000 ) ) ;
#30606=CARTESIAN_POINT ( 'NONE',  ( 12.18129165770028166, -1.906344006863165630, 232.6627636338612888 ) ) ;
#30620=CARTESIAN_POINT ( 'NONE',  ( -28.49999999970000175, 7.466149641070000342, 229.0000000000000000 ) ) ;
#30645=CARTESIAN_POINT ( 'NONE',  ( 2.382250895449999906, 11.80689512960000087, 231.9999989789999972 ) ) ;
#30660=CARTESIAN_POINT ( 'NONE',  ( -23.51354662350000169, -14.83147814589999847, 224.7915671760000009 ) ) ;
#30675=CARTESIAN_POINT ( 'NONE',  ( -27.04041630550000264, -9.934689828449998927, 230.6999999999999886 ) ) ;
#30681=CARTESIAN_POINT ( 'NONE',  ( -24.07583586439999834, -13.90018868249999962, 223.9000014189999774 ) ) ;
#30684=DIRECTION ( 'NONE',  ( 0.9002473904559572526, -0.4353787270609801308, 0.000000000000000000 ) ) ;
#30699=CARTESIAN_POINT ( 'NONE',  ( -1.089818731940000118, -28.47945802909999813, 224.6898005070000011 ) ) ;
#30701=CARTESIAN_POINT ( 'NONE',  ( -27.79999999999999716, -2.360778239559999931E-11, 229.0000000000000000 ) ) ;
#30709=FACE_OUTER_BOUND ( 'NONE', #12360, .T. ) ;
#30740=CARTESIAN_POINT ( 'NONE',  ( 27.53132593009999951, 1.219291334560000045E-11, 229.7313259299999686 ) ) ;
#30743=CARTESIAN_POINT ( 'NONE',  ( -23.11028700030000138, -15.72531859329999726, 222.0000000000000000 ) ) ;
#30755=CARTESIAN_POINT ( 'NONE',  ( 26.05511440549999946, -14.93230011260000012, 222.0000000000000000 ) ) ;
#30763=CARTESIAN_POINT ( 'NONE',  ( 26.95545383900000047, 8.667969224290001051, 229.0000000000000000 ) ) ;
#30780=CARTESIAN_POINT ( 'NONE',  ( 20.30405755279999980, 20.00000000000000000, 229.0000000000000000 ) ) ;
#30783=ADVANCED_FACE ( 'NONE', ( #16557 ), #17070, .F. ) ;
#30784=B_SPLINE_SURFACE_WITH_KNOTS ( 'NONE', 5, 1, ( 
 ( #5888, #1032 ),
 ( #15495, #10935 ),
 ( #6049, #10621 ),
 ( #20216, #25099 ),
 ( #3532, #22736 ),
 ( #13127, #15646 ),
 ( #25257, #30755 ),
 ( #23213, #16272 ),
 ( #25731, #30454 ) ),
 .UNSPECIFIED., .F., .F., .F.,
 ( 6, 3, 6 ),
 ( 2, 2 ),
 ( 0.000000000000000000, 55.31395627319999875, 94.75474476520000167 ),
 ( -3.500000000000000000, 3.500000000000000000 ),
 .UNSPECIFIED. ) ;
#30785=UNCERTAINTY_MEASURE_WITH_UNIT (LENGTH_MEASURE( 1.000000000000000082E-05 ), #28244, 'distance_accuracy_value', 'NONE');
#30791=CARTESIAN_POINT ( 'NONE',  ( 24.66410523950000311, -14.28055064019999953, 226.1000014189999945 ) ) ;
#30798=CARTESIAN_POINT ( 'NONE',  ( 23.56856306074712037, -14.74329105725733946, 225.4958374175672304 ) ) ;
#30820=CARTESIAN_POINT ( 'NONE',  ( -21.02335142420000125, 19.26967309480000168, 226.0000000000000000 ) ) ;
#30825=CARTESIAN_POINT ( 'NONE',  ( -23.69119896560000171, -20.94188573509999785, 229.2404163060000144 ) ) ;
#30826=ORIENTED_EDGE ( 'NONE', *, *, #8126, .T. ) ;
#30827=CARTESIAN_POINT ( 'NONE',  ( -24.15901410609999900, -15.12012600329999934, 224.4928788709999878 ) ) ;
#30846=B_SPLINE_CURVE_WITH_KNOTS ( 'NONE', 5,
 ( #6161, #21546, #13401, #16809, #14466, #1461 ),
 .UNSPECIFIED., .F., .F.,
 ( 6, 6 ),
 ( 64.89339659389999326, 88.69760957229999576 ),
 .UNSPECIFIED. ) ;
#30853=CARTESIAN_POINT ( 'NONE',  ( -0.6685465369699999938, -28.49273882800000024, 224.0990923460000204 ) ) ;
#30856=FACE_OUTER_BOUND ( 'NONE', #18287, .T. ) ;
#30861=EDGE_CURVE ( 'NONE', #21756, #28017, #3952, .T. ) ;
#30877=CARTESIAN_POINT ( 'NONE',  ( -24.55841378230000061, -14.46270012129999927, 226.0798679369999888 ) ) ;
#30883=CARTESIAN_POINT ( 'NONE',  ( -21.32009893540000078, 17.08474177209999922, 230.0000000000000000 ) ) ;
#30887=ORIENTED_EDGE ( 'NONE', *, *, #21740, .T. ) ;
#30893=ORIENTED_EDGE ( 'NONE', *, *, #3749, .T. ) ;
#30901=CARTESIAN_POINT ( 'NONE',  ( 27.24857305730000334, 4.341416115490000300E-12, 229.9172022069999741 ) ) ;
#30904=CARTESIAN_POINT ( 'NONE',  ( 28.01995124469999965, -5.907569749770000378, 222.0000000000000000 ) ) ;
#30910=CARTESIAN_POINT ( 'NONE',  ( 2.131628207279999844E-14, -1.704192342799999938E-14, 231.6999999999999886 ) ) ;
#30911=CARTESIAN_POINT ( 'NONE',  ( 11.49589634081054434, 4.456723487524678617, 232.6627635931969280 ) ) ;
#30916=CARTESIAN_POINT ( 'NONE',  ( -23.61125025500000163, 15.96150951279999930, 222.0000000000000000 ) ) ;
#30938=VERTEX_POINT ( 'NONE', #5373 ) ;
#30949=CARTESIAN_POINT ( 'NONE',  ( 20.25363919059999773, 20.00000851029999893, 229.3819260790000101 ) ) ;
#30952=CARTESIAN_POINT ( 'NONE',  ( -1.100001419170000050, -27.77850706310000106, 225.0000014190000002 ) ) ;
#30960=VERTEX_POINT ( 'NONE', #15279 ) ;
#30964=CARTESIAN_POINT ( 'NONE',  ( -24.34159889609999894, -14.82483853620000147, 224.0986003170000060 ) ) ;
#30975=CARTESIAN_POINT ( 'NONE',  ( 0.4086195922400000513, -12.10538642919999930, 231.9999991140000191 ) ) ;
#30979=CARTESIAN_POINT ( 'NONE',  ( -28.45771199730000234, 1.065814103639999922E-14, 229.4982322489999831 ) ) ;
#30981=CARTESIAN_POINT ( 'NONE',  ( -24.68204616399999907, -14.25020164319999871, 223.9000014189999774 ) ) ;
#31016=CARTESIAN_POINT ( 'NONE',  ( -19.99487511799999950, 20.00000620269999985, 229.8488538259999814 ) ) ;
#31040=CARTESIAN_POINT ( 'NONE',  ( 25.08428924680000094, -13.52916357279999993, 225.7601281139999969 ) ) ;
#31046=EDGE_LOOP ( 'NONE', ( #26738, #22180, #12719, #379 ) ) ;
#31056=CARTESIAN_POINT ( 'NONE',  ( 28.46656763489999875, -1.746773142929999967, 222.0000000000000000 ) ) ;
#31102=CARTESIAN_POINT ( 'NONE',  ( 18.92330595649999836, 19.72869720889999812, 229.8506619570000282 ) ) ;
#31103=CARTESIAN_POINT ( 'NONE',  ( -25.27355175290000133, 12.75978488059999805, 222.0000000000000000 ) ) ;
#31105=CARTESIAN_POINT ( 'NONE',  ( -0.1058797546490000130, -28.50006311429999784, 226.0959516479999820 ) ) ;
#31108=CARTESIAN_POINT ( 'NONE',  ( 24.00345430277922887, -14.02483715947875176, 226.1000014189999661 ) ) ;
#31110=B_SPLINE_SURFACE_WITH_KNOTS ( 'NONE', 5, 1, ( 
 ( #4607, #9487 ),
 ( #23817, #2414 ),
 ( #21610, #24124 ),
 ( #2563, #2265 ),
 ( #21761, #209 ),
 ( #9800, #28988 ),
 ( #17031, #22537 ),
 ( #14988, #29451 ),
 ( #5224, #5381 ) ),
 .UNSPECIFIED., .F., .F., .F.,
 ( 6, 3, 6 ),
 ( 2, 2 ),
 ( 0.000000000000000000, 55.31395511720000258, 94.75474465359999954 ),
 ( -3.500000000000000000, 3.500000000000000000 ),
 .UNSPECIFIED. ) ;
#31112=CARTESIAN_POINT ( 'NONE',  ( -26.80000000000000071, -7.283063041539999493E-14, 230.0000000000000000 ) ) ;
ENDSEC;
END-ISO-10303-21;
